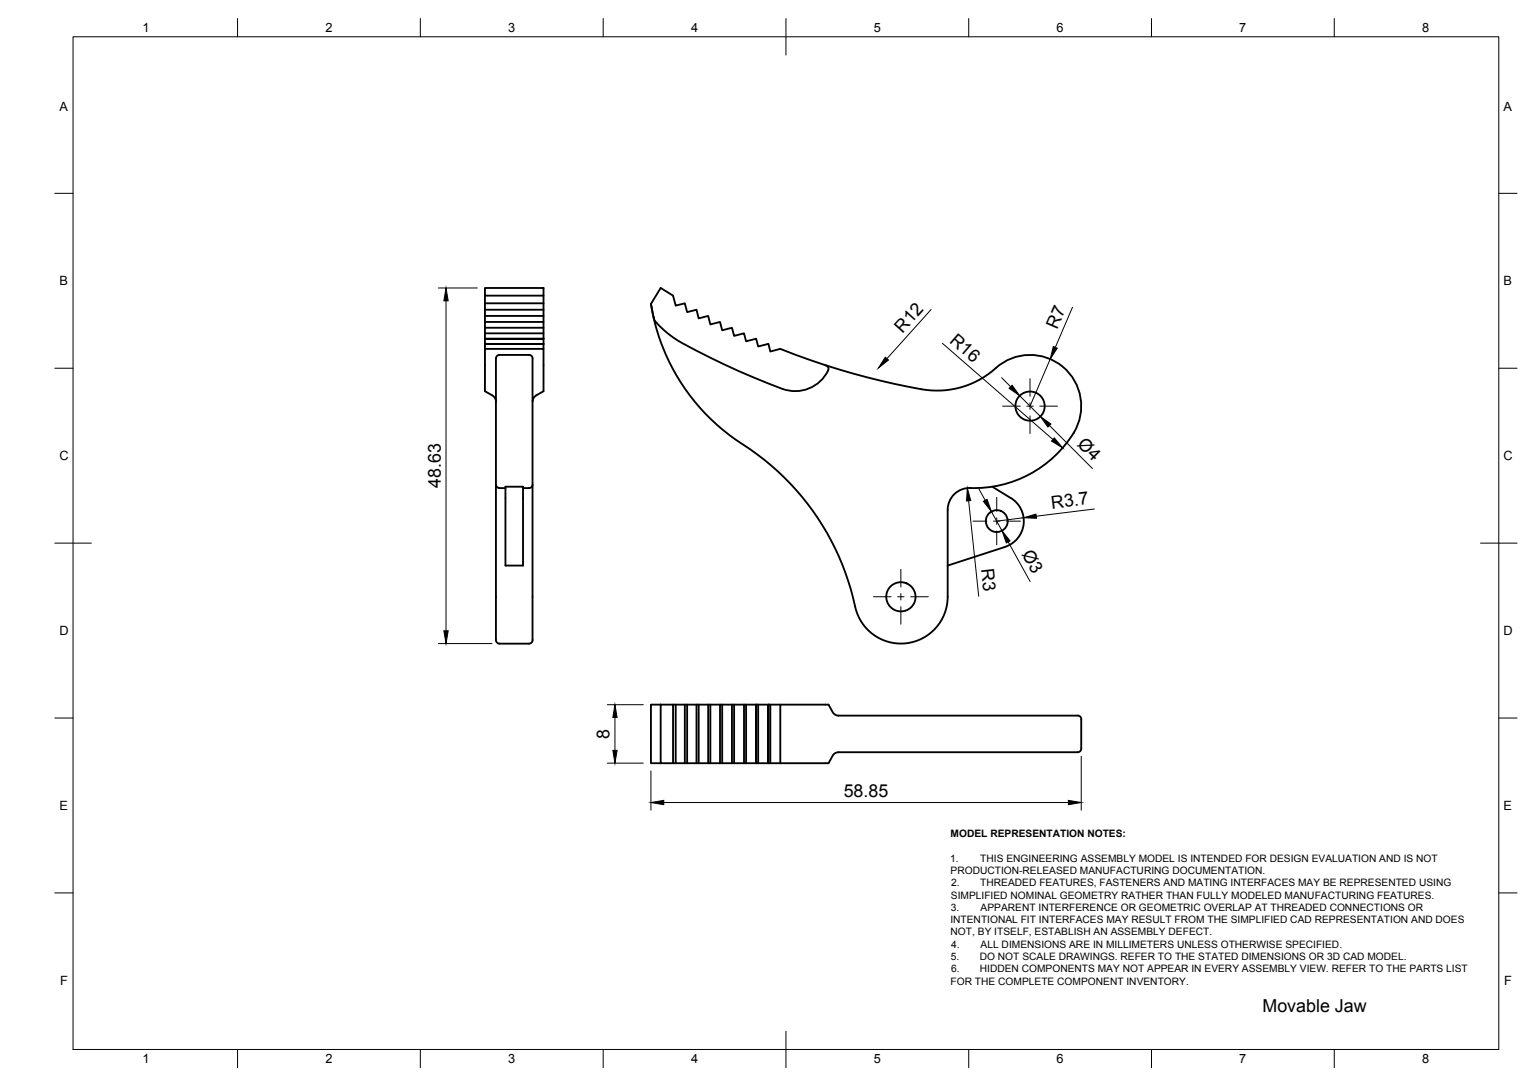
ISO-10303-21;
HEADER;
/* Generated by software containing ST-Developer
 * from STEP Tools, Inc. (www.steptools.com) 
 */

FILE_DESCRIPTION(
/* description */ ('STEP AP214'),
/* implementation_level */ '2;1');

FILE_NAME(
/* name */ 'Movable Jaw.step',
/* time_stamp */ '2026-10-06T11:11:25-07:00',
/* author */ (''),
/* organization */ (''),
/* preprocessor_version */ 'ST-DEVELOPER v20.2',
/* originating_system */ 'Autodesk Translation Framework v15.15.0.0',
/* authorisation */ '');

FILE_SCHEMA (('AUTOMOTIVE_DESIGN { 1 0 10303 214 3 1 1 }'));
ENDSEC;

DATA;
#10=MECHANICAL_DESIGN_GEOMETRIC_PRESENTATION_REPRESENTATION('',(#704),#47717);
#111=ELLIPSE('',#9597,55.9999994580806,27.9999998645779);
#112=ELLIPSE('',#9600,56.0000011433114,28.0000002857322);
#142=CONICAL_SURFACE('',#9608,105.,0.5235987755983);
#143=CONICAL_SURFACE('',#9610,13.5459216391339,0.5235987755983);
#144=CONICAL_SURFACE('',#9612,5.,0.5235987755983);
#145=CONICAL_SURFACE('',#9615,5.,0.5235987755983);
#146=CONICAL_SURFACE('',#9620,13.5459216391339,0.5235987755983);
#147=CONICAL_SURFACE('',#9622,105.,0.5235987755983);
#453=B_SPLINE_CURVE_WITH_KNOTS('',3,(#44399,#44400,#44401,#44402,#44403,
#44404,#44405,#44406,#44407,#44408,#44409,#44410,#44411,#44412,#44413,#44414,
#44415,#44416,#44417,#44418,#44419,#44420,#44421,#44422,#44423,#44424,#44425,
#44426,#44427,#44428,#44429,#44430,#44431,#44432,#44433,#44434,#44435,#44436,
#44437,#44438,#44439,#44440,#44441),.UNSPECIFIED.,.F.,.F.,(4,3,3,3,3,3,
3,3,3,3,3,3,3,3,4),(0.,0.000265218733424361,0.000529943392799562,0.000791311297886273,
0.00104485851075797,0.00120949425781351,0.00140442813951922,0.00159510196316745,
0.00177939478496708,0.00181424138672026,0.00194996928456625,0.00208057934802266,
0.00220782711137267,0.00232952375057779,0.00241898851562701),
 .UNSPECIFIED.);
#454=B_SPLINE_CURVE_WITH_KNOTS('',3,(#44450,#44451,#44452,#44453,#44454,
#44455,#44456,#44457),.UNSPECIFIED.,.F.,.F.,(4,2,2,4),(1.10972417955536E-15,
0.000601563815809569,0.00120312763161803,0.00240625526323496),
 .UNSPECIFIED.);
#455=B_SPLINE_CURVE_WITH_KNOTS('',3,(#44486,#44487,#44488,#44489,#44490,
#44491,#44492,#44493,#44494,#44495,#44496,#44497,#44498,#44499,#44500,#44501,
#44502,#44503,#44504,#44505,#44506,#44507,#44508,#44509,#44510,#44511,#44512,
#44513,#44514,#44515,#44516,#44517,#44518,#44519,#44520,#44521,#44522,#44523,
#44524,#44525),.UNSPECIFIED.,.F.,.F.,(4,3,3,3,3,3,3,3,3,3,3,3,3,4),(0.,
0.000120731756906386,0.000244724286038655,0.000330382072298398,0.00038742395842631,
0.000451543376039767,0.000587355431077626,0.000736422494620045,0.000783140574770168,
0.0007839342580256,0.00111532596981935,0.00117471086215525,0.00117522277660967,
0.00156628114954034),.UNSPECIFIED.);
#456=B_SPLINE_CURVE_WITH_KNOTS('',3,(#44533,#44534,#44535,#44536,#44537,
#44538,#44539,#44540,#44541,#44542,#44543,#44544,#44545,#44546,#44547,#44548,
#44549,#44550,#44551,#44552,#44553,#44554,#44555,#44556,#44557,#44558,#44559,
#44560,#44561,#44562,#44563,#44564,#44565,#44566,#44567,#44568,#44569),
 .UNSPECIFIED.,.F.,.F.,(4,3,3,3,3,3,3,3,3,3,3,3,4),(0.,0.000121030957133445,
0.000244083459183201,0.000368145253824231,0.000391521746120079,0.000542549206905392,
0.000692240215942904,0.000782245350403997,0.000783043492240158,0.0011402076544283,
0.00117391722717013,0.00117456523836024,0.00156608698448032),
 .UNSPECIFIED.);
#457=B_SPLINE_CURVE_WITH_KNOTS('',3,(#44678,#44679,#44680,#44681,#44682,
#44683,#44684),.UNSPECIFIED.,.F.,.F.,(4,3,4),(8.8191888018214E-12,0.00104225234663735,
0.00196541786057149),.UNSPECIFIED.);
#458=B_SPLINE_CURVE_WITH_KNOTS('',3,(#44686,#44687,#44688,#44689,#44690,
#44691,#44692,#44693,#44694,#44695,#44696,#44697,#44698,#44699,#44700,#44701,
#44702,#44703,#44704,#44705,#44706,#44707,#44708,#44709,#44710,#44711,#44712,
#44713,#44714,#44715,#44716),.UNSPECIFIED.,.F.,.F.,(4,3,3,3,3,3,3,3,3,3,
4),(0.,0.000282229008902596,0.000596615472147253,0.000672888082078944,0.000674913983482446,
0.00113908191323505,0.0013477148488729,0.00134982796696489,0.00185411344461373,
0.00236801844152055,0.00269965593392979),.UNSPECIFIED.);
#459=B_SPLINE_CURVE_WITH_KNOTS('',3,(#44724,#44725,#44726,#44727,#44728,
#44729,#44730,#44731,#44732,#44733,#44734,#44735,#44736,#44737,#44738,#44739,
#44740,#44741,#44742,#44743,#44744,#44745,#44746,#44747,#44748,#44749,#44750,
#44751),.UNSPECIFIED.,.F.,.F.,(4,3,3,3,3,3,3,3,3,4),(0.,0.000683898970964164,
0.00134585328061937,0.00134792532155823,0.00179669833308319,0.00201877992092906,
0.0020208379703943,0.00232967550949865,0.00260160458154724,0.00269170656123875),
 .UNSPECIFIED.);
#460=B_SPLINE_CURVE_WITH_KNOTS('',3,(#44753,#44754,#44755,#44756,#44757,
#44758,#44759),.UNSPECIFIED.,.F.,.F.,(4,3,4),(1.55158384577955E-17,0.00104225233782226,
0.0019654178517479),.UNSPECIFIED.);
#461=B_SPLINE_CURVE_WITH_KNOTS('',3,(#44766,#44767,#44768,#44769,#44770,
#44771,#44772,#44773,#44774,#44775,#44776,#44777),.UNSPECIFIED.,.F.,.F.,
(4,2,2,2,2,4),(0.,0.023927482322817,0.0451601219442732,0.0651153892897719,
0.0785588651844482,0.0909362631271192),.UNSPECIFIED.);
#462=B_SPLINE_CURVE_WITH_KNOTS('',3,(#44785,#44786,#44787,#44788,#44789,
#44790),.UNSPECIFIED.,.F.,.F.,(4,2,4),(1.03628274237769E-6,0.0204474690808872,
0.0408541618075523),.UNSPECIFIED.);
#463=B_SPLINE_CURVE_WITH_KNOTS('',3,(#44831,#44832,#44833,#44834),
 .UNSPECIFIED.,.F.,.F.,(4,4),(0.,0.00159208620889079),.UNSPECIFIED.);
#464=B_SPLINE_CURVE_WITH_KNOTS('',3,(#44836,#44837,#44838,#44839,#44840,
#44841),.UNSPECIFIED.,.F.,.F.,(4,2,4),(-0.0108288738373355,-0.00541184520716738,
0.),.UNSPECIFIED.);
#465=B_SPLINE_CURVE_WITH_KNOTS('',3,(#44857,#44858,#44859,#44860,#44861,
#44862),.UNSPECIFIED.,.F.,.F.,(4,2,4),(-0.0108279843969241,-0.00541695432919009,
-7.41619925991033E-7),.UNSPECIFIED.);
#466=B_SPLINE_CURVE_WITH_KNOTS('',3,(#44868,#44869,#44870,#44871),
 .UNSPECIFIED.,.F.,.F.,(4,4),(1.72172026516128E-9,0.00159208793060872),
 .UNSPECIFIED.);
#467=B_SPLINE_CURVE_WITH_KNOTS('',3,(#44877,#44878,#44879,#44880,#44881,
#44882,#44883,#44884,#44885,#44886,#44887,#44888),.UNSPECIFIED.,.F.,.F.,
(4,2,2,2,2,4),(-0.0909372297788789,-0.0786310994776589,-0.0652694224322856,
-0.0453380124663928,-0.0241275039307517,0.),.UNSPECIFIED.);
#468=B_SPLINE_CURVE_WITH_KNOTS('',3,(#44922,#44923,#44924,#44925,#44926,
#44927),.UNSPECIFIED.,.F.,.F.,(4,2,4),(-0.0408541865438099,-0.0204437555046671,
-1.03628388816493E-6),.UNSPECIFIED.);
#469=B_SPLINE_CURVE_WITH_KNOTS('',3,(#44929,#44930,#44931,#44932,#44933,
#44934,#44935,#44936,#44937,#44938,#44939,#44940,#44941,#44942,#44943,#44944,
#44945,#44946,#44947,#44948,#44949,#44950,#44951,#44952,#44953,#44954,#44955,
#44956,#44957,#44958,#44959,#44960,#44961,#44962),.UNSPECIFIED.,.F.,.F.,
(4,3,3,3,3,3,3,3,3,3,3,4),(0.,0.000262944884148408,0.000263234297577755,
0.000494857606554129,0.000525889768296816,0.000526476175615979,0.00064121097647369,
0.000757086494550119,0.000788834652445224,0.000880494124966269,0.000970158609493951,
0.00105177953659363),.UNSPECIFIED.);
#470=B_SPLINE_CURVE_WITH_KNOTS('',3,(#44966,#44967,#44968,#44969,#44970,
#44971,#44972,#44973,#44974,#44975,#44976,#44977,#44978,#44979,#44980,#44981,
#44982,#44983,#44984,#44985,#44986,#44987,#44988,#44989,#44990,#44991,#44992,
#44993,#44994,#44995,#44996,#44997,#44998,#44999,#45000,#45001,#45002),
 .UNSPECIFIED.,.F.,.F.,(4,3,3,3,3,3,3,3,3,3,3,3,4),(0.,0.000244362774360397,
0.000262384380603159,0.000262964527186242,0.000497872683618592,0.0005253349756591,
0.000525929054372485,0.000639225228153213,0.000753740945662581,0.000788893581558727,
0.000881307299681151,0.000971994008335542,0.00105185810874497),
 .UNSPECIFIED.);
#590=(
BOUNDED_SURFACE()
B_SPLINE_SURFACE(3,2,((#45068,#45069,#45070),(#45071,#45072,#45073),(#45074,
#45075,#45076),(#45077,#45078,#45079),(#45080,#45081,#45082),(#45083,#45084,
#45085),(#45086,#45087,#45088),(#45089,#45090,#45091)),.UNSPECIFIED.,.F.,
 .F.,.F.)
B_SPLINE_SURFACE_WITH_KNOTS((4,2,2,4),(3,3),(-0.000265671039808014,0.000664177599544138,
0.00132835519908425,0.00292238143798051),(-0.000697566251991853,1.),
 .UNSPECIFIED.)
GEOMETRIC_REPRESENTATION_ITEM()
RATIONAL_B_SPLINE_SURFACE(((1.00006735358899,0.951722442998278,1.),(1.00009085795633,
0.934875034398606,1.),(1.00011995255585,0.914020671505109,1.),(1.00017679132716,
0.873279902332299,1.),(1.000202236158,0.855041612592702,1.),(1.00029314270923,
0.789881815244371,1.),(1.00036608854593,0.737595859260726,1.),(1.00044993425484,
0.677497116903894,1.)))
REPRESENTATION_ITEM('')
SURFACE()
);
#591=(
BOUNDED_SURFACE()
B_SPLINE_SURFACE(3,2,((#45093,#45094,#45095),(#45096,#45097,#45098),(#45099,
#45100,#45101),(#45102,#45103,#45104)),.UNSPECIFIED.,.F.,.F.,.F.)
B_SPLINE_SURFACE_WITH_KNOTS((4,4),(3,3),(1.73472347597681E-18,0.00194751686681009),
(0.,1.),.UNSPECIFIED.)
GEOMETRIC_REPRESENTATION_ITEM()
RATIONAL_B_SPLINE_SURFACE(((1.,0.9363704575632,1.),(1.,0.937911573932337,
1.),(1.,0.939551224752395,1.),(1.,0.941276432107511,1.)))
REPRESENTATION_ITEM('')
SURFACE()
);
#592=(
BOUNDED_SURFACE()
B_SPLINE_SURFACE(3,2,((#45115,#45116,#45117),(#45118,#45119,#45120),(#45121,
#45122,#45123),(#45124,#45125,#45126),(#45127,#45128,#45129),(#45130,#45131,
#45132),(#45133,#45134,#45135),(#45136,#45137,#45138)),.UNSPECIFIED.,.F.,
 .F.,.F.)
B_SPLINE_SURFACE_WITH_KNOTS((4,2,2,4),(3,3),(-0.000264848297699882,0.00132424148849942,
0.00198636223274913,0.00291333127469873),(-0.000376747913465724,1.),
 .UNSPECIFIED.)
GEOMETRIC_REPRESENTATION_ITEM()
RATIONAL_B_SPLINE_SURFACE(((1.00024295987203,0.677556446441725,1.),(1.00019753111789,
0.73784709770907,1.),(1.00015862247899,0.789484595236775,1.),(1.00010910533939,
0.855201136507422,1.),(1.00009527454653,0.873556636784662,1.),(1.00006486797912,
0.91391063254542,1.),(1.00004913297578,0.934793300746539,1.),(1.0000362266027,
0.951921959744005,1.)))
REPRESENTATION_ITEM('')
SURFACE()
);
#593=(
BOUNDED_SURFACE()
B_SPLINE_SURFACE(3,2,((#45140,#45141,#45142),(#45143,#45144,#45145),(#45146,
#45147,#45148),(#45149,#45150,#45151)),.UNSPECIFIED.,.F.,.F.,.F.)
B_SPLINE_SURFACE_WITH_KNOTS((4,4),(3,3),(-3.46944695195361E-18,0.00194751686680595),
(0.,1.),.UNSPECIFIED.)
GEOMETRIC_REPRESENTATION_ITEM()
RATIONAL_B_SPLINE_SURFACE(((1.,0.936370457563209,1.),(1.,0.937911573932344,
1.),(1.,0.939551224752402,1.),(1.,0.941276432107508,1.)))
REPRESENTATION_ITEM('')
SURFACE()
);
#594=(
BOUNDED_SURFACE()
B_SPLINE_SURFACE(3,2,((#45152,#45153,#45154),(#45155,#45156,#45157),(#45158,
#45159,#45160),(#45161,#45162,#45163)),.UNSPECIFIED.,.F.,.F.,.F.)
B_SPLINE_SURFACE_WITH_KNOTS((4,4),(3,3),(-8.67361737988404E-19,0.00145502531726256),
(0.,1.),.UNSPECIFIED.)
GEOMETRIC_REPRESENTATION_ITEM()
RATIONAL_B_SPLINE_SURFACE(((1.,0.668532680377463,1.),(1.,0.667444009600454,
1.),(1.,0.666151431295988,1.),(1.,0.66453110293118,1.)))
REPRESENTATION_ITEM('')
SURFACE()
);
#595=(
BOUNDED_SURFACE()
B_SPLINE_SURFACE(3,2,((#45165,#45166,#45167),(#45168,#45169,#45170),(#45171,
#45172,#45173),(#45174,#45175,#45176),(#45177,#45178,#45179),(#45180,#45181,
#45182),(#45183,#45184,#45185),(#45186,#45187,#45188)),.UNSPECIFIED.,.F.,
 .F.,.F.)
B_SPLINE_SURFACE_WITH_KNOTS((4,2,2,4),(3,3),(-8.23993651088983E-18,0.000785858548320119,
0.00117878782248018,0.00157171709664025),(0.,1.),.UNSPECIFIED.)
GEOMETRIC_REPRESENTATION_ITEM()
RATIONAL_B_SPLINE_SURFACE(((1.,0.707106781186552,1.),(1.,0.700392709855563,
1.),(1.,0.693103478140052,1.),(1.,0.68292873029758,1.),(1.,0.679593975234355,
1.),(1.,0.673572573507934,1.),(1.,0.670859596930162,1.),(1.,0.668532680377463,
1.)))
REPRESENTATION_ITEM('')
SURFACE()
);
#596=(
BOUNDED_SURFACE()
B_SPLINE_SURFACE(3,2,((#45208,#45209,#45210),(#45211,#45212,#45213),(#45214,
#45215,#45216),(#45217,#45218,#45219),(#45220,#45221,#45222),(#45223,#45224,
#45225),(#45226,#45227,#45228),(#45229,#45230,#45231)),.UNSPECIFIED.,.F.,
 .F.,.F.)
B_SPLINE_SURFACE_WITH_KNOTS((4,2,2,4),(3,3),(-1.25767452008319E-17,0.000785889192074472,
0.00117883378811171,0.00157177838414896),(0.,1.),.UNSPECIFIED.)
GEOMETRIC_REPRESENTATION_ITEM()
RATIONAL_B_SPLINE_SURFACE(((1.,0.668532680377451,1.),(1.,0.673123216892149,
1.),(1.,0.679555858731309,1.),(1.,0.68973495589728,1.),(1.,0.693295125056467,
1.),(1.,0.700263684314459,1.),(1.,0.703699964289598,1.),(1.,0.707106781186548,
1.)))
REPRESENTATION_ITEM('')
SURFACE()
);
#597=(
BOUNDED_SURFACE()
B_SPLINE_SURFACE(3,2,((#45233,#45234,#45235),(#45236,#45237,#45238),(#45239,
#45240,#45241),(#45242,#45243,#45244)),.UNSPECIFIED.,.F.,.F.,.F.)
B_SPLINE_SURFACE_WITH_KNOTS((4,4),(3,3),(-8.67361737988404E-19,0.00145502531726205),
(0.,1.),.UNSPECIFIED.)
GEOMETRIC_REPRESENTATION_ITEM()
RATIONAL_B_SPLINE_SURFACE(((1.,0.668532680377451,1.),(1.,0.667444009600447,
1.),(1.,0.666151431295967,1.),(1.,0.664531102931197,1.)))
REPRESENTATION_ITEM('')
SURFACE()
);
#630=TOROIDAL_SURFACE('',#9516,5.9,0.5);
#631=TOROIDAL_SURFACE('',#9521,5.9,0.5);
#632=TOROIDAL_SURFACE('',#9535,14.989297312108,1.);
#633=TOROIDAL_SURFACE('',#9539,14.989297312108,1.);
#634=TOROIDAL_SURFACE('',#9626,6.44337567297407,1.);
#635=TOROIDAL_SURFACE('',#9628,106.443375672974,1.);
#636=TOROIDAL_SURFACE('',#9629,6.44337567297407,1.);
#637=TOROIDAL_SURFACE('',#9631,106.443375672974,1.);
#638=TOROIDAL_SURFACE('',#9660,15.5,0.5);
#639=TOROIDAL_SURFACE('',#9663,3.5,0.5);
#640=TOROIDAL_SURFACE('',#9666,35.5,0.5);
#641=TOROIDAL_SURFACE('',#9668,27.5,0.5);
#642=TOROIDAL_SURFACE('',#9671,15.5,0.5);
#643=TOROIDAL_SURFACE('',#9674,3.5,0.5);
#644=TOROIDAL_SURFACE('',#9677,35.5,0.5);
#645=TOROIDAL_SURFACE('',#9679,27.5,0.5);
#646=TOROIDAL_SURFACE('',#9684,100.5,0.5);
#647=TOROIDAL_SURFACE('',#9686,12.5,0.5);
#648=TOROIDAL_SURFACE('',#9688,6.5,0.5);
#649=TOROIDAL_SURFACE('',#9696,6.5,0.5);
#650=TOROIDAL_SURFACE('',#9698,12.5,0.5);
#651=TOROIDAL_SURFACE('',#9700,100.5,0.5);
#680=SHAPE_REPRESENTATION_RELATIONSHIP('SRR','None',#47767,#692);
#692=ADVANCED_BREP_SHAPE_REPRESENTATION('',(#716),#47711);
#704=STYLED_ITEM('',(#47830),#716);
#716=MANIFOLD_SOLID_BREP('Body1',#8931);
#731=FACE_BOUND('',#2898,.T.);
#732=FACE_BOUND('',#2899,.T.);
#733=FACE_BOUND('',#2901,.T.);
#734=FACE_BOUND('',#2902,.T.);
#735=FACE_BOUND('',#2927,.T.);
#736=FACE_BOUND('',#2929,.T.);
#812=PLANE('',#9563);
#813=PLANE('',#9573);
#814=PLANE('',#9583);
#815=PLANE('',#9595);
#816=PLANE('',#9604);
#817=PLANE('',#9611);
#818=PLANE('',#9619);
#819=PLANE('',#9625);
#820=PLANE('',#9635);
#821=PLANE('',#9636);
#822=PLANE('',#9638);
#823=PLANE('',#9641);
#824=PLANE('',#9642);
#825=PLANE('',#9643);
#826=PLANE('',#9644);
#827=PLANE('',#9645);
#828=PLANE('',#9646);
#829=PLANE('',#9647);
#830=PLANE('',#9648);
#831=PLANE('',#9649);
#832=PLANE('',#9650);
#833=PLANE('',#9651);
#834=PLANE('',#9652);
#835=PLANE('',#9653);
#836=PLANE('',#9654);
#837=PLANE('',#9655);
#838=PLANE('',#9656);
#839=PLANE('',#9657);
#840=PLANE('',#9658);
#841=PLANE('',#9659);
#1146=LINE('',#44377,#1633);
#1147=LINE('',#44383,#1634);
#1148=LINE('',#44389,#1635);
#1149=LINE('',#44463,#1636);
#1150=LINE('',#44466,#1637);
#1151=LINE('',#44468,#1638);
#1152=LINE('',#44469,#1639);
#1153=LINE('',#44475,#1640);
#1154=LINE('',#44478,#1641);
#1155=LINE('',#44529,#1642);
#1156=LINE('',#44574,#1643);
#1157=LINE('',#44580,#1644);
#1158=LINE('',#44583,#1645);
#1159=LINE('',#44587,#1646);
#1160=LINE('',#44591,#1647);
#1161=LINE('',#44606,#1648);
#1162=LINE('',#44622,#1649);
#1163=LINE('',#44632,#1650);
#1164=LINE('',#44634,#1651);
#1165=LINE('',#44636,#1652);
#1166=LINE('',#44638,#1653);
#1167=LINE('',#44640,#1654);
#1168=LINE('',#44641,#1655);
#1169=LINE('',#44646,#1656);
#1170=LINE('',#44650,#1657);
#1171=LINE('',#44654,#1658);
#1172=LINE('',#44659,#1659);
#1173=LINE('',#44663,#1660);
#1174=LINE('',#44670,#1661);
#1175=LINE('',#44672,#1662);
#1176=LINE('',#44673,#1663);
#1177=LINE('',#44720,#1664);
#1178=LINE('',#44791,#1665);
#1179=LINE('',#44793,#1666);
#1180=LINE('',#44795,#1667);
#1181=LINE('',#44797,#1668);
#1182=LINE('',#44799,#1669);
#1183=LINE('',#44801,#1670);
#1184=LINE('',#44803,#1671);
#1185=LINE('',#44805,#1672);
#1186=LINE('',#44807,#1673);
#1187=LINE('',#44809,#1674);
#1188=LINE('',#44811,#1675);
#1189=LINE('',#44813,#1676);
#1190=LINE('',#44815,#1677);
#1191=LINE('',#44817,#1678);
#1192=LINE('',#44818,#1679);
#1193=LINE('',#44820,#1680);
#1194=LINE('',#44821,#1681);
#1195=LINE('',#44823,#1682);
#1196=LINE('',#44824,#1683);
#1197=LINE('',#44827,#1684);
#1198=LINE('',#44829,#1685);
#1199=LINE('',#44854,#1686);
#1200=LINE('',#44863,#1687);
#1201=LINE('',#44872,#1688);
#1202=LINE('',#44890,#1689);
#1203=LINE('',#44891,#1690);
#1204=LINE('',#44893,#1691);
#1205=LINE('',#44894,#1692);
#1206=LINE('',#44896,#1693);
#1207=LINE('',#44898,#1694);
#1208=LINE('',#44900,#1695);
#1209=LINE('',#44902,#1696);
#1210=LINE('',#44904,#1697);
#1211=LINE('',#44906,#1698);
#1212=LINE('',#44908,#1699);
#1213=LINE('',#44910,#1700);
#1214=LINE('',#44912,#1701);
#1215=LINE('',#44914,#1702);
#1216=LINE('',#44916,#1703);
#1217=LINE('',#44918,#1704);
#1218=LINE('',#44920,#1705);
#1219=LINE('',#44921,#1706);
#1220=LINE('',#45010,#1707);
#1221=LINE('',#45012,#1708);
#1222=LINE('',#45013,#1709);
#1223=LINE('',#45016,#1710);
#1224=LINE('',#45021,#1711);
#1225=LINE('',#45023,#1712);
#1226=LINE('',#45026,#1713);
#1227=LINE('',#45027,#1714);
#1228=LINE('',#45030,#1715);
#1229=LINE('',#45032,#1716);
#1230=LINE('',#45033,#1717);
#1231=LINE('',#45035,#1718);
#1232=LINE('',#45036,#1719);
#1233=LINE('',#45038,#1720);
#1234=LINE('',#45039,#1721);
#1235=LINE('',#45041,#1722);
#1236=LINE('',#45042,#1723);
#1237=LINE('',#45044,#1724);
#1238=LINE('',#45045,#1725);
#1239=LINE('',#45053,#1726);
#1240=LINE('',#45056,#1727);
#1633=VECTOR('',#11135,1.5);
#1634=VECTOR('',#11142,2.00000000000001);
#1635=VECTOR('',#11149,2.);
#1636=VECTOR('',#11172,1000.);
#1637=VECTOR('',#11175,1000.);
#1638=VECTOR('',#11178,1000.);
#1639=VECTOR('',#11179,1000.);
#1640=VECTOR('',#11184,1000.);
#1641=VECTOR('',#11187,1000.);
#1642=VECTOR('',#11196,1000.);
#1643=VECTOR('',#11203,1000.);
#1644=VECTOR('',#11208,1000.);
#1645=VECTOR('',#11211,1000.);
#1646=VECTOR('',#11214,1000.);
#1647=VECTOR('',#11217,1000.);
#1648=VECTOR('',#11234,1000.);
#1649=VECTOR('',#11251,1000.);
#1650=VECTOR('',#11264,1000.);
#1651=VECTOR('',#11265,1000.);
#1652=VECTOR('',#11266,1000.);
#1653=VECTOR('',#11267,1000.);
#1654=VECTOR('',#11268,1000.);
#1655=VECTOR('',#11269,1000.);
#1656=VECTOR('',#11274,1000.);
#1657=VECTOR('',#11277,1000.);
#1658=VECTOR('',#11280,1000.);
#1659=VECTOR('',#11285,1000.);
#1660=VECTOR('',#11288,1000.);
#1661=VECTOR('',#11299,1000.);
#1662=VECTOR('',#11300,1000.);
#1663=VECTOR('',#11301,1000.);
#1664=VECTOR('',#11308,1000.);
#1665=VECTOR('',#11327,1000.);
#1666=VECTOR('',#11328,1000.);
#1667=VECTOR('',#11329,1000.);
#1668=VECTOR('',#11330,1000.);
#1669=VECTOR('',#11331,1000.);
#1670=VECTOR('',#11332,1000.);
#1671=VECTOR('',#11333,1000.);
#1672=VECTOR('',#11334,1000.);
#1673=VECTOR('',#11335,1000.);
#1674=VECTOR('',#11336,1000.);
#1675=VECTOR('',#11337,1000.);
#1676=VECTOR('',#11338,1000.);
#1677=VECTOR('',#11339,1000.);
#1678=VECTOR('',#11340,1000.);
#1679=VECTOR('',#11341,1000.);
#1680=VECTOR('',#11342,1000.);
#1681=VECTOR('',#11343,1000.);
#1682=VECTOR('',#11344,1000.);
#1683=VECTOR('',#11345,1000.);
#1684=VECTOR('',#11348,1000.);
#1685=VECTOR('',#11351,1000.);
#1686=VECTOR('',#11370,1000.);
#1687=VECTOR('',#11373,1000.);
#1688=VECTOR('',#11378,1000.);
#1689=VECTOR('',#11387,1000.);
#1690=VECTOR('',#11388,1000.);
#1691=VECTOR('',#11389,1000.);
#1692=VECTOR('',#11390,1000.);
#1693=VECTOR('',#11391,1000.);
#1694=VECTOR('',#11392,1000.);
#1695=VECTOR('',#11393,1000.);
#1696=VECTOR('',#11394,1000.);
#1697=VECTOR('',#11395,1000.);
#1698=VECTOR('',#11396,1000.);
#1699=VECTOR('',#11397,1000.);
#1700=VECTOR('',#11398,1000.);
#1701=VECTOR('',#11399,1000.);
#1702=VECTOR('',#11400,1000.);
#1703=VECTOR('',#11401,1000.);
#1704=VECTOR('',#11402,1000.);
#1705=VECTOR('',#11403,1000.);
#1706=VECTOR('',#11404,1000.);
#1707=VECTOR('',#11425,1000.);
#1708=VECTOR('',#11426,1000.);
#1709=VECTOR('',#11427,1000.);
#1710=VECTOR('',#11430,1000.);
#1711=VECTOR('',#11437,1000.);
#1712=VECTOR('',#11440,1000.);
#1713=VECTOR('',#11445,1000.);
#1714=VECTOR('',#11446,1000.);
#1715=VECTOR('',#11451,1000.);
#1716=VECTOR('',#11454,1000.);
#1717=VECTOR('',#11455,1000.);
#1718=VECTOR('',#11458,1000.);
#1719=VECTOR('',#11459,1000.);
#1720=VECTOR('',#11462,1000.);
#1721=VECTOR('',#11463,1000.);
#1722=VECTOR('',#11466,1000.);
#1723=VECTOR('',#11467,1000.);
#1724=VECTOR('',#11470,1000.);
#1725=VECTOR('',#11471,1000.);
#1726=VECTOR('',#11486,1000.);
#1727=VECTOR('',#11491,1000.);
#1998=CYLINDRICAL_SURFACE('',#9526,1.5);
#1999=CYLINDRICAL_SURFACE('',#9529,2.00000000000001);
#2000=CYLINDRICAL_SURFACE('',#9532,2.);
#2001=CYLINDRICAL_SURFACE('',#9543,100.);
#2002=CYLINDRICAL_SURFACE('',#9546,6.4);
#2003=CYLINDRICAL_SURFACE('',#9547,100.);
#2004=CYLINDRICAL_SURFACE('',#9550,100.);
#2005=CYLINDRICAL_SURFACE('',#9557,100.);
#2006=CYLINDRICAL_SURFACE('',#9560,3.);
#2007=CYLINDRICAL_SURFACE('',#9584,16.);
#2008=CYLINDRICAL_SURFACE('',#9589,7.);
#2009=CYLINDRICAL_SURFACE('',#9592,12.);
#2010=CYLINDRICAL_SURFACE('',#9596,28.);
#2011=CYLINDRICAL_SURFACE('',#9601,35.);
#2012=CYLINDRICAL_SURFACE('',#9632,3.);
#2013=CYLINDRICAL_SURFACE('',#9640,3.7);
#2014=CYLINDRICAL_SURFACE('',#9665,0.500000000000001);
#2015=CYLINDRICAL_SURFACE('',#9676,0.500000000000001);
#2016=CYLINDRICAL_SURFACE('',#9692,0.499999999999999);
#2363=FACE_OUTER_BOUND('',#2884,.T.);
#2364=FACE_OUTER_BOUND('',#2885,.T.);
#2365=FACE_OUTER_BOUND('',#2886,.T.);
#2366=FACE_OUTER_BOUND('',#2887,.T.);
#2367=FACE_OUTER_BOUND('',#2888,.T.);
#2368=FACE_OUTER_BOUND('',#2889,.T.);
#2369=FACE_OUTER_BOUND('',#2890,.T.);
#2370=FACE_OUTER_BOUND('',#2891,.T.);
#2371=FACE_OUTER_BOUND('',#2892,.T.);
#2372=FACE_OUTER_BOUND('',#2893,.T.);
#2373=FACE_OUTER_BOUND('',#2894,.T.);
#2374=FACE_OUTER_BOUND('',#2895,.T.);
#2375=FACE_OUTER_BOUND('',#2896,.T.);
#2376=FACE_OUTER_BOUND('',#2897,.T.);
#2377=FACE_OUTER_BOUND('',#2900,.T.);
#2378=FACE_OUTER_BOUND('',#2903,.T.);
#2379=FACE_OUTER_BOUND('',#2904,.T.);
#2380=FACE_OUTER_BOUND('',#2905,.T.);
#2381=FACE_OUTER_BOUND('',#2906,.T.);
#2382=FACE_OUTER_BOUND('',#2907,.T.);
#2383=FACE_OUTER_BOUND('',#2908,.T.);
#2384=FACE_OUTER_BOUND('',#2909,.T.);
#2385=FACE_OUTER_BOUND('',#2910,.T.);
#2386=FACE_OUTER_BOUND('',#2911,.T.);
#2387=FACE_OUTER_BOUND('',#2912,.T.);
#2388=FACE_OUTER_BOUND('',#2913,.T.);
#2389=FACE_OUTER_BOUND('',#2914,.T.);
#2390=FACE_OUTER_BOUND('',#2915,.T.);
#2391=FACE_OUTER_BOUND('',#2916,.T.);
#2392=FACE_OUTER_BOUND('',#2917,.T.);
#2393=FACE_OUTER_BOUND('',#2918,.T.);
#2394=FACE_OUTER_BOUND('',#2919,.T.);
#2395=FACE_OUTER_BOUND('',#2920,.T.);
#2396=FACE_OUTER_BOUND('',#2921,.T.);
#2397=FACE_OUTER_BOUND('',#2922,.T.);
#2398=FACE_OUTER_BOUND('',#2923,.T.);
#2399=FACE_OUTER_BOUND('',#2924,.T.);
#2400=FACE_OUTER_BOUND('',#2925,.T.);
#2401=FACE_OUTER_BOUND('',#2926,.T.);
#2402=FACE_OUTER_BOUND('',#2928,.T.);
#2403=FACE_OUTER_BOUND('',#2930,.T.);
#2404=FACE_OUTER_BOUND('',#2931,.T.);
#2405=FACE_OUTER_BOUND('',#2932,.T.);
#2406=FACE_OUTER_BOUND('',#2933,.T.);
#2407=FACE_OUTER_BOUND('',#2934,.T.);
#2408=FACE_OUTER_BOUND('',#2935,.T.);
#2409=FACE_OUTER_BOUND('',#2936,.T.);
#2410=FACE_OUTER_BOUND('',#2937,.T.);
#2411=FACE_OUTER_BOUND('',#2938,.T.);
#2412=FACE_OUTER_BOUND('',#2939,.T.);
#2413=FACE_OUTER_BOUND('',#2940,.T.);
#2414=FACE_OUTER_BOUND('',#2941,.T.);
#2415=FACE_OUTER_BOUND('',#2942,.T.);
#2416=FACE_OUTER_BOUND('',#2943,.T.);
#2417=FACE_OUTER_BOUND('',#2944,.T.);
#2418=FACE_OUTER_BOUND('',#2945,.T.);
#2419=FACE_OUTER_BOUND('',#2946,.T.);
#2420=FACE_OUTER_BOUND('',#2947,.T.);
#2421=FACE_OUTER_BOUND('',#2948,.T.);
#2422=FACE_OUTER_BOUND('',#2949,.T.);
#2423=FACE_OUTER_BOUND('',#2950,.T.);
#2424=FACE_OUTER_BOUND('',#2951,.T.);
#2425=FACE_OUTER_BOUND('',#2952,.T.);
#2426=FACE_OUTER_BOUND('',#2953,.T.);
#2427=FACE_OUTER_BOUND('',#2954,.T.);
#2428=FACE_OUTER_BOUND('',#2955,.T.);
#2429=FACE_OUTER_BOUND('',#2956,.T.);
#2430=FACE_OUTER_BOUND('',#2957,.T.);
#2431=FACE_OUTER_BOUND('',#2958,.T.);
#2432=FACE_OUTER_BOUND('',#2959,.T.);
#2433=FACE_OUTER_BOUND('',#2960,.T.);
#2434=FACE_OUTER_BOUND('',#2961,.T.);
#2435=FACE_OUTER_BOUND('',#2962,.T.);
#2436=FACE_OUTER_BOUND('',#2963,.T.);
#2437=FACE_OUTER_BOUND('',#2964,.T.);
#2438=FACE_OUTER_BOUND('',#2965,.T.);
#2439=FACE_OUTER_BOUND('',#2966,.T.);
#2440=FACE_OUTER_BOUND('',#2967,.T.);
#2441=FACE_OUTER_BOUND('',#2968,.T.);
#2442=FACE_OUTER_BOUND('',#2969,.T.);
#2443=FACE_OUTER_BOUND('',#2970,.T.);
#2444=FACE_OUTER_BOUND('',#2971,.T.);
#2445=FACE_OUTER_BOUND('',#2972,.T.);
#2446=FACE_OUTER_BOUND('',#2973,.T.);
#2447=FACE_OUTER_BOUND('',#2974,.T.);
#2448=FACE_OUTER_BOUND('',#2975,.T.);
#2449=FACE_OUTER_BOUND('',#2976,.T.);
#2884=EDGE_LOOP('',(#7347,#7348,#7349,#7350));
#2885=EDGE_LOOP('',(#7351,#7352,#7353,#7354));
#2886=EDGE_LOOP('',(#7355,#7356,#7357,#7358));
#2887=EDGE_LOOP('',(#7359,#7360,#7361,#7362));
#2888=EDGE_LOOP('',(#7363,#7364,#7365,#7366));
#2889=EDGE_LOOP('',(#7367,#7368,#7369,#7370));
#2890=EDGE_LOOP('',(#7371,#7372,#7373,#7374));
#2891=EDGE_LOOP('',(#7375,#7376,#7377,#7378));
#2892=EDGE_LOOP('',(#7379,#7380,#7381,#7382));
#2893=EDGE_LOOP('',(#7383,#7384,#7385,#7386));
#2894=EDGE_LOOP('',(#7387,#7388,#7389,#7390,#7391,#7392,#7393,#7394,#7395,
#7396));
#2895=EDGE_LOOP('',(#7397,#7398,#7399,#7400));
#2896=EDGE_LOOP('',(#7401,#7402,#7403,#7404));
#2897=EDGE_LOOP('',(#7405,#7406,#7407,#7408,#7409,#7410,#7411,#7412,#7413,
#7414,#7415,#7416));
#2898=EDGE_LOOP('',(#7417));
#2899=EDGE_LOOP('',(#7418));
#2900=EDGE_LOOP('',(#7419,#7420,#7421,#7422,#7423,#7424,#7425,#7426,#7427,
#7428,#7429,#7430));
#2901=EDGE_LOOP('',(#7431));
#2902=EDGE_LOOP('',(#7432));
#2903=EDGE_LOOP('',(#7433,#7434,#7435,#7436,#7437,#7438,#7439,#7440));
#2904=EDGE_LOOP('',(#7441,#7442,#7443,#7444,#7445,#7446,#7447,#7448));
#2905=EDGE_LOOP('',(#7449,#7450,#7451,#7452));
#2906=EDGE_LOOP('',(#7453,#7454,#7455,#7456));
#2907=EDGE_LOOP('',(#7457,#7458,#7459,#7460));
#2908=EDGE_LOOP('',(#7461,#7462,#7463,#7464,#7465,#7466,#7467,#7468,#7469,
#7470));
#2909=EDGE_LOOP('',(#7471,#7472,#7473,#7474));
#2910=EDGE_LOOP('',(#7475,#7476,#7477,#7478,#7479,#7480,#7481,#7482,#7483,
#7484,#7485,#7486,#7487,#7488,#7489,#7490,#7491,#7492,#7493,#7494,#7495,
#7496,#7497,#7498,#7499,#7500,#7501,#7502,#7503));
#2911=EDGE_LOOP('',(#7504,#7505,#7506,#7507));
#2912=EDGE_LOOP('',(#7508,#7509,#7510,#7511));
#2913=EDGE_LOOP('',(#7512,#7513,#7514));
#2914=EDGE_LOOP('',(#7515,#7516,#7517,#7518));
#2915=EDGE_LOOP('',(#7519,#7520,#7521,#7522));
#2916=EDGE_LOOP('',(#7523,#7524,#7525));
#2917=EDGE_LOOP('',(#7526,#7527,#7528,#7529));
#2918=EDGE_LOOP('',(#7530,#7531,#7532,#7533));
#2919=EDGE_LOOP('',(#7534,#7535,#7536,#7537,#7538,#7539,#7540,#7541,#7542,
#7543,#7544,#7545,#7546,#7547,#7548,#7549,#7550,#7551,#7552,#7553,#7554,
#7555,#7556,#7557,#7558,#7559,#7560,#7561,#7562));
#2920=EDGE_LOOP('',(#7563,#7564,#7565,#7566));
#2921=EDGE_LOOP('',(#7567,#7568,#7569,#7570));
#2922=EDGE_LOOP('',(#7571,#7572,#7573,#7574));
#2923=EDGE_LOOP('',(#7575,#7576,#7577,#7578));
#2924=EDGE_LOOP('',(#7579,#7580,#7581,#7582));
#2925=EDGE_LOOP('',(#7583,#7584,#7585,#7586));
#2926=EDGE_LOOP('',(#7587,#7588,#7589,#7590,#7591,#7592));
#2927=EDGE_LOOP('',(#7593));
#2928=EDGE_LOOP('',(#7594,#7595,#7596,#7597,#7598,#7599));
#2929=EDGE_LOOP('',(#7600));
#2930=EDGE_LOOP('',(#7601,#7602,#7603,#7604));
#2931=EDGE_LOOP('',(#7605,#7606,#7607,#7608));
#2932=EDGE_LOOP('',(#7609,#7610,#7611,#7612));
#2933=EDGE_LOOP('',(#7613,#7614,#7615,#7616));
#2934=EDGE_LOOP('',(#7617,#7618,#7619,#7620));
#2935=EDGE_LOOP('',(#7621,#7622,#7623,#7624));
#2936=EDGE_LOOP('',(#7625,#7626,#7627,#7628));
#2937=EDGE_LOOP('',(#7629,#7630,#7631,#7632));
#2938=EDGE_LOOP('',(#7633,#7634,#7635,#7636));
#2939=EDGE_LOOP('',(#7637,#7638,#7639,#7640));
#2940=EDGE_LOOP('',(#7641,#7642,#7643,#7644));
#2941=EDGE_LOOP('',(#7645,#7646,#7647,#7648));
#2942=EDGE_LOOP('',(#7649,#7650,#7651,#7652));
#2943=EDGE_LOOP('',(#7653,#7654,#7655,#7656));
#2944=EDGE_LOOP('',(#7657,#7658,#7659,#7660));
#2945=EDGE_LOOP('',(#7661,#7662,#7663,#7664));
#2946=EDGE_LOOP('',(#7665,#7666,#7667,#7668));
#2947=EDGE_LOOP('',(#7669,#7670,#7671,#7672));
#2948=EDGE_LOOP('',(#7673,#7674,#7675,#7676));
#2949=EDGE_LOOP('',(#7677,#7678,#7679,#7680));
#2950=EDGE_LOOP('',(#7681,#7682,#7683,#7684));
#2951=EDGE_LOOP('',(#7685,#7686,#7687,#7688));
#2952=EDGE_LOOP('',(#7689,#7690,#7691,#7692));
#2953=EDGE_LOOP('',(#7693,#7694,#7695,#7696));
#2954=EDGE_LOOP('',(#7697,#7698,#7699,#7700));
#2955=EDGE_LOOP('',(#7701,#7702,#7703,#7704));
#2956=EDGE_LOOP('',(#7705,#7706,#7707,#7708,#7709));
#2957=EDGE_LOOP('',(#7710,#7711,#7712,#7713));
#2958=EDGE_LOOP('',(#7714,#7715,#7716,#7717));
#2959=EDGE_LOOP('',(#7718,#7719,#7720,#7721));
#2960=EDGE_LOOP('',(#7722,#7723,#7724,#7725));
#2961=EDGE_LOOP('',(#7726,#7727,#7728,#7729));
#2962=EDGE_LOOP('',(#7730,#7731,#7732,#7733));
#2963=EDGE_LOOP('',(#7734,#7735,#7736,#7737,#7738));
#2964=EDGE_LOOP('',(#7739,#7740,#7741,#7742));
#2965=EDGE_LOOP('',(#7743,#7744,#7745,#7746));
#2966=EDGE_LOOP('',(#7747,#7748,#7749,#7750));
#2967=EDGE_LOOP('',(#7751,#7752,#7753,#7754));
#2968=EDGE_LOOP('',(#7755,#7756,#7757,#7758));
#2969=EDGE_LOOP('',(#7759,#7760,#7761));
#2970=EDGE_LOOP('',(#7762,#7763,#7764,#7765));
#2971=EDGE_LOOP('',(#7766,#7767,#7768));
#2972=EDGE_LOOP('',(#7769,#7770,#7771,#7772));
#2973=EDGE_LOOP('',(#7773,#7774,#7775,#7776));
#2974=EDGE_LOOP('',(#7777,#7778,#7779,#7780));
#2975=EDGE_LOOP('',(#7781,#7782,#7783,#7784));
#2976=EDGE_LOOP('',(#7785,#7786,#7787,#7788));
#3314=CIRCLE('',#9517,5.9);
#3315=CIRCLE('',#9518,0.500000000000001);
#3316=CIRCLE('',#9519,6.4);
#3317=CIRCLE('',#9520,0.500000000000001);
#3318=CIRCLE('',#9522,6.4);
#3319=CIRCLE('',#9523,0.500000000000001);
#3320=CIRCLE('',#9524,5.9);
#3321=CIRCLE('',#9525,0.500000000000001);
#3322=CIRCLE('',#9527,1.5);
#3323=CIRCLE('',#9528,1.5);
#3324=CIRCLE('',#9530,2.00000000000001);
#3325=CIRCLE('',#9531,2.00000000000001);
#3326=CIRCLE('',#9533,2.);
#3327=CIRCLE('',#9534,2.);
#3328=CIRCLE('',#9536,14.1232719083235);
#3329=CIRCLE('',#9537,1.);
#3330=CIRCLE('',#9538,14.989297312108);
#3331=CIRCLE('',#9540,14.989297312108);
#3332=CIRCLE('',#9541,1.);
#3333=CIRCLE('',#9542,14.1232719083235);
#3334=CIRCLE('',#9544,100.);
#3335=CIRCLE('',#9545,100.);
#3336=CIRCLE('',#9548,100.);
#3337=CIRCLE('',#9549,100.);
#3338=CIRCLE('',#9551,100.);
#3339=CIRCLE('',#9552,390.917804157437);
#3340=CIRCLE('',#9553,100.);
#3341=CIRCLE('',#9554,100.);
#3342=CIRCLE('',#9555,390.917804135939);
#3343=CIRCLE('',#9556,100.);
#3344=CIRCLE('',#9558,100.);
#3345=CIRCLE('',#9559,100.);
#3346=CIRCLE('',#9561,3.);
#3347=CIRCLE('',#9562,3.);
#3348=CIRCLE('',#9564,12.5);
#3349=CIRCLE('',#9565,100.5);
#3350=CIRCLE('',#9566,6.44337567297407);
#3351=CIRCLE('',#9567,106.443375672974);
#3352=CIRCLE('',#9568,27.5);
#3353=CIRCLE('',#9569,35.5);
#3354=CIRCLE('',#9570,3.5);
#3355=CIRCLE('',#9571,15.5);
#3356=CIRCLE('',#9572,6.50000000000001);
#3357=CIRCLE('',#9574,12.5);
#3358=CIRCLE('',#9575,6.50000000000001);
#3359=CIRCLE('',#9576,15.5);
#3360=CIRCLE('',#9577,3.5);
#3361=CIRCLE('',#9578,35.5);
#3362=CIRCLE('',#9579,27.5);
#3363=CIRCLE('',#9580,106.443375672974);
#3364=CIRCLE('',#9581,6.44337567297407);
#3365=CIRCLE('',#9582,100.5);
#3366=CIRCLE('',#9585,16.);
#3367=CIRCLE('',#9586,16.);
#3368=CIRCLE('',#9587,16.);
#3369=CIRCLE('',#9588,16.);
#3370=CIRCLE('',#9590,7.);
#3371=CIRCLE('',#9591,7.);
#3372=CIRCLE('',#9593,12.);
#3373=CIRCLE('',#9594,12.);
#3374=CIRCLE('',#9598,28.);
#3375=CIRCLE('',#9599,28.);
#3376=CIRCLE('',#9602,35.);
#3377=CIRCLE('',#9603,35.);
#3378=CIRCLE('',#9605,5.);
#3379=CIRCLE('',#9606,105.);
#3380=CIRCLE('',#9607,13.5459216391339);
#3381=CIRCLE('',#9609,105.57735026919);
#3382=CIRCLE('',#9613,601.835963345588);
#3383=CIRCLE('',#9614,5.57735026918963);
#3384=CIRCLE('',#9616,5.57735026918963);
#3385=CIRCLE('',#9617,601.835963357857);
#3386=CIRCLE('',#9618,5.);
#3387=CIRCLE('',#9621,13.5459216391339);
#3388=CIRCLE('',#9623,105.57735026919);
#3389=CIRCLE('',#9624,105.);
#3390=CIRCLE('',#9627,0.999999999999998);
#3391=CIRCLE('',#9630,0.999999999999998);
#3392=CIRCLE('',#9633,3.);
#3393=CIRCLE('',#9634,3.);
#3394=CIRCLE('',#9637,3.7);
#3395=CIRCLE('',#9639,3.7);
#3396=CIRCLE('',#9661,0.5);
#3397=CIRCLE('',#9662,0.500000000000001);
#3398=CIRCLE('',#9664,0.500000000000001);
#3399=CIRCLE('',#9667,0.500000000000003);
#3400=CIRCLE('',#9669,0.499999999999998);
#3401=CIRCLE('',#9670,0.500000000000005);
#3402=CIRCLE('',#9672,0.5);
#3403=CIRCLE('',#9673,0.500000000000001);
#3404=CIRCLE('',#9675,0.500000000000001);
#3405=CIRCLE('',#9678,0.500000000000003);
#3406=CIRCLE('',#9680,0.499999999999998);
#3407=CIRCLE('',#9681,0.499999999999992);
#3408=CIRCLE('',#9682,0.500000000000009);
#3409=CIRCLE('',#9683,0.499999999999998);
#3410=CIRCLE('',#9685,0.499999999999998);
#3411=CIRCLE('',#9687,0.5);
#3412=CIRCLE('',#9689,0.5);
#3413=CIRCLE('',#9691,0.499999999999999);
#3414=CIRCLE('',#9693,0.499999999999999);
#3415=CIRCLE('',#9695,0.5);
#3416=CIRCLE('',#9697,0.5);
#3417=CIRCLE('',#9699,0.499999999999998);
#3418=CIRCLE('',#9701,0.499999999999998);
#3419=CIRCLE('',#9702,0.500000000000009);
#4059=VERTEX_POINT('',#44356);
#4060=VERTEX_POINT('',#44357);
#4061=VERTEX_POINT('',#44359);
#4062=VERTEX_POINT('',#44361);
#4063=VERTEX_POINT('',#44365);
#4064=VERTEX_POINT('',#44366);
#4065=VERTEX_POINT('',#44368);
#4066=VERTEX_POINT('',#44370);
#4067=VERTEX_POINT('',#44374);
#4068=VERTEX_POINT('',#44376);
#4069=VERTEX_POINT('',#44380);
#4070=VERTEX_POINT('',#44382);
#4071=VERTEX_POINT('',#44386);
#4072=VERTEX_POINT('',#44388);
#4073=VERTEX_POINT('',#44392);
#4074=VERTEX_POINT('',#44393);
#4075=VERTEX_POINT('',#44395);
#4076=VERTEX_POINT('',#44397);
#4077=VERTEX_POINT('',#44443);
#4078=VERTEX_POINT('',#44444);
#4079=VERTEX_POINT('',#44446);
#4080=VERTEX_POINT('',#44448);
#4081=VERTEX_POINT('',#44459);
#4082=VERTEX_POINT('',#44460);
#4083=VERTEX_POINT('',#44462);
#4084=VERTEX_POINT('',#44464);
#4085=VERTEX_POINT('',#44471);
#4086=VERTEX_POINT('',#44472);
#4087=VERTEX_POINT('',#44474);
#4088=VERTEX_POINT('',#44476);
#4089=VERTEX_POINT('',#44480);
#4090=VERTEX_POINT('',#44481);
#4091=VERTEX_POINT('',#44483);
#4092=VERTEX_POINT('',#44485);
#4093=VERTEX_POINT('',#44526);
#4094=VERTEX_POINT('',#44528);
#4095=VERTEX_POINT('',#44530);
#4096=VERTEX_POINT('',#44532);
#4097=VERTEX_POINT('',#44570);
#4098=VERTEX_POINT('',#44572);
#4099=VERTEX_POINT('',#44576);
#4100=VERTEX_POINT('',#44577);
#4101=VERTEX_POINT('',#44579);
#4102=VERTEX_POINT('',#44581);
#4103=VERTEX_POINT('',#44585);
#4104=VERTEX_POINT('',#44586);
#4105=VERTEX_POINT('',#44588);
#4106=VERTEX_POINT('',#44590);
#4107=VERTEX_POINT('',#44594);
#4108=VERTEX_POINT('',#44595);
#4109=VERTEX_POINT('',#44597);
#4110=VERTEX_POINT('',#44599);
#4111=VERTEX_POINT('',#44602);
#4112=VERTEX_POINT('',#44605);
#4113=VERTEX_POINT('',#44607);
#4114=VERTEX_POINT('',#44609);
#4115=VERTEX_POINT('',#44613);
#4116=VERTEX_POINT('',#44614);
#4117=VERTEX_POINT('',#44616);
#4118=VERTEX_POINT('',#44618);
#4119=VERTEX_POINT('',#44620);
#4120=VERTEX_POINT('',#44623);
#4121=VERTEX_POINT('',#44626);
#4122=VERTEX_POINT('',#44628);
#4123=VERTEX_POINT('',#44633);
#4124=VERTEX_POINT('',#44635);
#4125=VERTEX_POINT('',#44637);
#4126=VERTEX_POINT('',#44639);
#4127=VERTEX_POINT('',#44643);
#4128=VERTEX_POINT('',#44645);
#4129=VERTEX_POINT('',#44647);
#4130=VERTEX_POINT('',#44649);
#4131=VERTEX_POINT('',#44651);
#4132=VERTEX_POINT('',#44653);
#4133=VERTEX_POINT('',#44657);
#4134=VERTEX_POINT('',#44658);
#4135=VERTEX_POINT('',#44660);
#4136=VERTEX_POINT('',#44662);
#4137=VERTEX_POINT('',#44669);
#4138=VERTEX_POINT('',#44671);
#4139=VERTEX_POINT('',#44675);
#4140=VERTEX_POINT('',#44677);
#4141=VERTEX_POINT('',#44685);
#4142=VERTEX_POINT('',#44717);
#4143=VERTEX_POINT('',#44719);
#4144=VERTEX_POINT('',#44721);
#4145=VERTEX_POINT('',#44723);
#4146=VERTEX_POINT('',#44752);
#4147=VERTEX_POINT('',#44765);
#4148=VERTEX_POINT('',#44778);
#4149=VERTEX_POINT('',#44780);
#4150=VERTEX_POINT('',#44782);
#4151=VERTEX_POINT('',#44784);
#4152=VERTEX_POINT('',#44792);
#4153=VERTEX_POINT('',#44794);
#4154=VERTEX_POINT('',#44796);
#4155=VERTEX_POINT('',#44798);
#4156=VERTEX_POINT('',#44800);
#4157=VERTEX_POINT('',#44802);
#4158=VERTEX_POINT('',#44804);
#4159=VERTEX_POINT('',#44806);
#4160=VERTEX_POINT('',#44808);
#4161=VERTEX_POINT('',#44810);
#4162=VERTEX_POINT('',#44812);
#4163=VERTEX_POINT('',#44814);
#4164=VERTEX_POINT('',#44816);
#4165=VERTEX_POINT('',#44819);
#4166=VERTEX_POINT('',#44822);
#4167=VERTEX_POINT('',#44826);
#4168=VERTEX_POINT('',#44843);
#4169=VERTEX_POINT('',#44847);
#4170=VERTEX_POINT('',#44848);
#4171=VERTEX_POINT('',#44850);
#4172=VERTEX_POINT('',#44852);
#4173=VERTEX_POINT('',#44856);
#4174=VERTEX_POINT('',#44865);
#4175=VERTEX_POINT('',#44866);
#4176=VERTEX_POINT('',#44889);
#4177=VERTEX_POINT('',#44892);
#4178=VERTEX_POINT('',#44895);
#4179=VERTEX_POINT('',#44897);
#4180=VERTEX_POINT('',#44899);
#4181=VERTEX_POINT('',#44901);
#4182=VERTEX_POINT('',#44903);
#4183=VERTEX_POINT('',#44905);
#4184=VERTEX_POINT('',#44907);
#4185=VERTEX_POINT('',#44909);
#4186=VERTEX_POINT('',#44911);
#4187=VERTEX_POINT('',#44913);
#4188=VERTEX_POINT('',#44915);
#4189=VERTEX_POINT('',#44917);
#4190=VERTEX_POINT('',#44919);
#4191=VERTEX_POINT('',#45009);
#4192=VERTEX_POINT('',#45011);
#4193=VERTEX_POINT('',#45015);
#4194=VERTEX_POINT('',#45019);
#5199=EDGE_CURVE('',#4059,#4060,#3314,.T.);
#5200=EDGE_CURVE('',#4061,#4059,#3315,.T.);
#5201=EDGE_CURVE('',#4062,#4061,#3316,.T.);
#5202=EDGE_CURVE('',#4062,#4060,#3317,.T.);
#5203=EDGE_CURVE('',#4063,#4064,#3318,.T.);
#5204=EDGE_CURVE('',#4065,#4063,#3319,.T.);
#5205=EDGE_CURVE('',#4066,#4065,#3320,.T.);
#5206=EDGE_CURVE('',#4066,#4064,#3321,.T.);
#5207=EDGE_CURVE('',#4067,#4067,#3322,.T.);
#5208=EDGE_CURVE('',#4067,#4068,#1146,.T.);
#5209=EDGE_CURVE('',#4068,#4068,#3323,.T.);
#5210=EDGE_CURVE('',#4069,#4069,#3324,.T.);
#5211=EDGE_CURVE('',#4069,#4070,#1147,.T.);
#5212=EDGE_CURVE('',#4070,#4070,#3325,.T.);
#5213=EDGE_CURVE('',#4071,#4071,#3326,.T.);
#5214=EDGE_CURVE('',#4071,#4072,#1148,.T.);
#5215=EDGE_CURVE('',#4072,#4072,#3327,.T.);
#5216=EDGE_CURVE('',#4073,#4074,#3328,.T.);
#5217=EDGE_CURVE('',#4073,#4075,#3329,.T.);
#5218=EDGE_CURVE('',#4076,#4075,#3330,.T.);
#5219=EDGE_CURVE('',#4076,#4074,#453,.T.);
#5220=EDGE_CURVE('',#4077,#4078,#3331,.T.);
#5221=EDGE_CURVE('',#4077,#4079,#3332,.T.);
#5222=EDGE_CURVE('',#4080,#4079,#3333,.T.);
#5223=EDGE_CURVE('',#4080,#4078,#454,.T.);
#5224=EDGE_CURVE('',#4081,#4082,#3334,.T.);
#5225=EDGE_CURVE('',#4081,#4083,#1149,.T.);
#5226=EDGE_CURVE('',#4083,#4084,#3335,.T.);
#5227=EDGE_CURVE('',#4082,#4084,#1150,.T.);
#5228=EDGE_CURVE('',#4061,#4063,#1151,.T.);
#5229=EDGE_CURVE('',#4062,#4064,#1152,.T.);
#5230=EDGE_CURVE('',#4085,#4086,#3336,.T.);
#5231=EDGE_CURVE('',#4086,#4087,#1153,.T.);
#5232=EDGE_CURVE('',#4088,#4087,#3337,.T.);
#5233=EDGE_CURVE('',#4088,#4085,#1154,.T.);
#5234=EDGE_CURVE('',#4089,#4090,#3338,.T.);
#5235=EDGE_CURVE('',#4089,#4091,#3339,.T.);
#5236=EDGE_CURVE('',#4091,#4092,#455,.T.);
#5237=EDGE_CURVE('',#4092,#4093,#3340,.T.);
#5238=EDGE_CURVE('',#4093,#4094,#1155,.T.);
#5239=EDGE_CURVE('',#4094,#4095,#3341,.T.);
#5240=EDGE_CURVE('',#4095,#4096,#456,.T.);
#5241=EDGE_CURVE('',#4096,#4097,#3342,.T.);
#5242=EDGE_CURVE('',#4097,#4098,#3343,.T.);
#5243=EDGE_CURVE('',#4098,#4090,#1156,.T.);
#5244=EDGE_CURVE('',#4099,#4100,#3344,.T.);
#5245=EDGE_CURVE('',#4100,#4101,#1157,.T.);
#5246=EDGE_CURVE('',#4102,#4101,#3345,.T.);
#5247=EDGE_CURVE('',#4102,#4099,#1158,.T.);
#5248=EDGE_CURVE('',#4103,#4104,#1159,.T.);
#5249=EDGE_CURVE('',#4103,#4105,#3346,.T.);
#5250=EDGE_CURVE('',#4106,#4105,#1160,.T.);
#5251=EDGE_CURVE('',#4104,#4106,#3347,.T.);
#5252=EDGE_CURVE('',#4107,#4108,#3348,.T.);
#5253=EDGE_CURVE('',#4108,#4109,#3349,.T.);
#5254=EDGE_CURVE('',#4109,#4110,#3350,.T.);
#5255=EDGE_CURVE('',#4110,#4077,#3351,.T.);
#5256=EDGE_CURVE('',#4078,#4111,#3352,.T.);
#5257=EDGE_CURVE('',#4111,#4059,#3353,.T.);
#5258=EDGE_CURVE('',#4060,#4112,#1161,.T.);
#5259=EDGE_CURVE('',#4112,#4113,#3354,.T.);
#5260=EDGE_CURVE('',#4113,#4114,#3355,.T.);
#5261=EDGE_CURVE('',#4114,#4107,#3356,.T.);
#5262=EDGE_CURVE('',#4115,#4116,#3357,.T.);
#5263=EDGE_CURVE('',#4116,#4117,#3358,.T.);
#5264=EDGE_CURVE('',#4117,#4118,#3359,.T.);
#5265=EDGE_CURVE('',#4118,#4119,#3360,.T.);
#5266=EDGE_CURVE('',#4119,#4066,#1162,.T.);
#5267=EDGE_CURVE('',#4065,#4120,#3361,.T.);
#5268=EDGE_CURVE('',#4120,#4076,#3362,.T.);
#5269=EDGE_CURVE('',#4075,#4121,#3363,.T.);
#5270=EDGE_CURVE('',#4121,#4122,#3364,.T.);
#5271=EDGE_CURVE('',#4122,#4115,#3365,.T.);
#5272=EDGE_CURVE('',#4064,#4103,#1163,.T.);
#5273=EDGE_CURVE('',#4104,#4123,#1164,.T.);
#5274=EDGE_CURVE('',#4124,#4123,#1165,.T.);
#5275=EDGE_CURVE('',#4125,#4124,#1166,.T.);
#5276=EDGE_CURVE('',#4125,#4126,#1167,.T.);
#5277=EDGE_CURVE('',#4126,#4062,#1168,.T.);
#5278=EDGE_CURVE('',#4105,#4127,#3366,.T.);
#5279=EDGE_CURVE('',#4127,#4128,#1169,.T.);
#5280=EDGE_CURVE('',#4128,#4129,#3367,.T.);
#5281=EDGE_CURVE('',#4129,#4130,#1170,.T.);
#5282=EDGE_CURVE('',#4130,#4131,#3368,.T.);
#5283=EDGE_CURVE('',#4132,#4131,#1171,.T.);
#5284=EDGE_CURVE('',#4106,#4132,#3369,.T.);
#5285=EDGE_CURVE('',#4133,#4134,#1172,.T.);
#5286=EDGE_CURVE('',#4133,#4135,#3370,.T.);
#5287=EDGE_CURVE('',#4135,#4136,#1173,.T.);
#5288=EDGE_CURVE('',#4136,#4134,#3371,.T.);
#5289=EDGE_CURVE('',#4093,#4133,#3372,.T.);
#5290=EDGE_CURVE('',#4134,#4094,#3373,.T.);
#5291=EDGE_CURVE('',#4084,#4137,#1174,.T.);
#5292=EDGE_CURVE('',#4138,#4137,#1175,.T.);
#5293=EDGE_CURVE('',#4082,#4138,#1176,.T.);
#5294=EDGE_CURVE('',#4137,#4139,#111,.T.);
#5295=EDGE_CURVE('',#4139,#4140,#457,.T.);
#5296=EDGE_CURVE('',#4140,#4141,#458,.T.);
#5297=EDGE_CURVE('',#4141,#4142,#3374,.T.);
#5298=EDGE_CURVE('',#4143,#4142,#1177,.T.);
#5299=EDGE_CURVE('',#4143,#4144,#3375,.T.);
#5300=EDGE_CURVE('',#4144,#4145,#459,.T.);
#5301=EDGE_CURVE('',#4145,#4146,#460,.T.);
#5302=EDGE_CURVE('',#4138,#4146,#112,.T.);
#5303=EDGE_CURVE('',#4061,#4143,#3376,.T.);
#5304=EDGE_CURVE('',#4142,#4063,#3377,.T.);
#5305=EDGE_CURVE('',#4097,#4147,#461,.T.);
#5306=EDGE_CURVE('',#4147,#4148,#3378,.T.);
#5307=EDGE_CURVE('',#4149,#4148,#3379,.T.);
#5308=EDGE_CURVE('',#4150,#4149,#3380,.T.);
#5309=EDGE_CURVE('',#4150,#4151,#462,.T.);
#5310=EDGE_CURVE('',#4137,#4151,#1178,.T.);
#5311=EDGE_CURVE('',#4083,#4152,#1179,.T.);
#5312=EDGE_CURVE('',#4152,#4153,#1180,.T.);
#5313=EDGE_CURVE('',#4153,#4154,#1181,.T.);
#5314=EDGE_CURVE('',#4154,#4155,#1182,.T.);
#5315=EDGE_CURVE('',#4155,#4156,#1183,.T.);
#5316=EDGE_CURVE('',#4156,#4157,#1184,.T.);
#5317=EDGE_CURVE('',#4157,#4158,#1185,.T.);
#5318=EDGE_CURVE('',#4158,#4159,#1186,.T.);
#5319=EDGE_CURVE('',#4159,#4160,#1187,.T.);
#5320=EDGE_CURVE('',#4160,#4161,#1188,.T.);
#5321=EDGE_CURVE('',#4161,#4162,#1189,.T.);
#5322=EDGE_CURVE('',#4162,#4163,#1190,.T.);
#5323=EDGE_CURVE('',#4163,#4164,#1191,.T.);
#5324=EDGE_CURVE('',#4164,#4100,#1192,.T.);
#5325=EDGE_CURVE('',#4099,#4165,#1193,.T.);
#5326=EDGE_CURVE('',#4165,#4086,#1194,.T.);
#5327=EDGE_CURVE('',#4085,#4166,#1195,.T.);
#5328=EDGE_CURVE('',#4166,#4098,#1196,.T.);
#5329=EDGE_CURVE('',#4167,#4148,#1197,.T.);
#5330=EDGE_CURVE('',#4167,#4073,#3381,.T.);
#5331=EDGE_CURVE('',#4073,#4149,#1198,.T.);
#5332=EDGE_CURVE('',#4074,#4150,#463,.T.);
#5333=EDGE_CURVE('',#4151,#4139,#464,.T.);
#5334=EDGE_CURVE('',#4147,#4168,#3382,.T.);
#5335=EDGE_CURVE('',#4168,#4167,#3383,.T.);
#5336=EDGE_CURVE('',#4169,#4170,#3384,.T.);
#5337=EDGE_CURVE('',#4170,#4171,#3385,.T.);
#5338=EDGE_CURVE('',#4171,#4172,#3386,.T.);
#5339=EDGE_CURVE('',#4172,#4169,#1199,.T.);
#5340=EDGE_CURVE('',#4146,#4173,#465,.T.);
#5341=EDGE_CURVE('',#4138,#4173,#1200,.T.);
#5342=EDGE_CURVE('',#4174,#4175,#3387,.T.);
#5343=EDGE_CURVE('',#4174,#4080,#466,.T.);
#5344=EDGE_CURVE('',#4175,#4079,#1201,.T.);
#5345=EDGE_CURVE('',#4079,#4169,#3388,.T.);
#5346=EDGE_CURVE('',#4175,#4172,#3389,.T.);
#5347=EDGE_CURVE('',#4171,#4089,#467,.T.);
#5348=EDGE_CURVE('',#4176,#4090,#1202,.T.);
#5349=EDGE_CURVE('',#4088,#4176,#1203,.T.);
#5350=EDGE_CURVE('',#4177,#4087,#1204,.T.);
#5351=EDGE_CURVE('',#4102,#4177,#1205,.T.);
#5352=EDGE_CURVE('',#4178,#4101,#1206,.T.);
#5353=EDGE_CURVE('',#4179,#4178,#1207,.T.);
#5354=EDGE_CURVE('',#4180,#4179,#1208,.T.);
#5355=EDGE_CURVE('',#4181,#4180,#1209,.T.);
#5356=EDGE_CURVE('',#4182,#4181,#1210,.T.);
#5357=EDGE_CURVE('',#4183,#4182,#1211,.T.);
#5358=EDGE_CURVE('',#4184,#4183,#1212,.T.);
#5359=EDGE_CURVE('',#4185,#4184,#1213,.T.);
#5360=EDGE_CURVE('',#4186,#4185,#1214,.T.);
#5361=EDGE_CURVE('',#4187,#4186,#1215,.T.);
#5362=EDGE_CURVE('',#4188,#4187,#1216,.T.);
#5363=EDGE_CURVE('',#4189,#4188,#1217,.T.);
#5364=EDGE_CURVE('',#4190,#4189,#1218,.T.);
#5365=EDGE_CURVE('',#4081,#4190,#1219,.T.);
#5366=EDGE_CURVE('',#4173,#4174,#468,.T.);
#5367=EDGE_CURVE('',#4109,#4170,#469,.T.);
#5368=EDGE_CURVE('',#4110,#4169,#3390,.T.);
#5369=EDGE_CURVE('',#4168,#4122,#470,.T.);
#5370=EDGE_CURVE('',#4167,#4121,#3391,.T.);
#5371=EDGE_CURVE('',#4129,#4126,#3392,.T.);
#5372=EDGE_CURVE('',#4125,#4130,#3393,.T.);
#5373=EDGE_CURVE('',#4191,#4132,#1220,.T.);
#5374=EDGE_CURVE('',#4192,#4131,#1221,.T.);
#5375=EDGE_CURVE('',#4192,#4191,#1222,.T.);
#5376=EDGE_CURVE('',#4124,#4193,#1223,.T.);
#5377=EDGE_CURVE('',#4193,#4192,#3394,.T.);
#5378=EDGE_CURVE('',#4194,#4191,#3395,.T.);
#5379=EDGE_CURVE('',#4123,#4194,#1224,.T.);
#5380=EDGE_CURVE('',#4193,#4194,#1225,.T.);
#5381=EDGE_CURVE('',#4189,#4153,#1226,.T.);
#5382=EDGE_CURVE('',#4152,#4190,#1227,.T.);
#5383=EDGE_CURVE('',#4154,#4188,#1228,.T.);
#5384=EDGE_CURVE('',#4156,#4186,#1229,.T.);
#5385=EDGE_CURVE('',#4187,#4155,#1230,.T.);
#5386=EDGE_CURVE('',#4158,#4184,#1231,.T.);
#5387=EDGE_CURVE('',#4185,#4157,#1232,.T.);
#5388=EDGE_CURVE('',#4160,#4182,#1233,.T.);
#5389=EDGE_CURVE('',#4183,#4159,#1234,.T.);
#5390=EDGE_CURVE('',#4162,#4180,#1235,.T.);
#5391=EDGE_CURVE('',#4181,#4161,#1236,.T.);
#5392=EDGE_CURVE('',#4164,#4178,#1237,.T.);
#5393=EDGE_CURVE('',#4179,#4163,#1238,.T.);
#5394=EDGE_CURVE('',#4166,#4176,#1239,.T.);
#5395=EDGE_CURVE('',#4165,#4177,#1240,.T.);
#5396=EDGE_CURVE('',#4117,#4127,#3396,.T.);
#5397=EDGE_CURVE('',#4118,#4105,#3397,.T.);
#5398=EDGE_CURVE('',#4119,#4103,#3398,.T.);
#5399=EDGE_CURVE('',#4120,#4142,#3399,.T.);
#5400=EDGE_CURVE('',#4076,#4141,#3400,.T.);
#5401=EDGE_CURVE('',#4074,#4140,#3401,.T.);
#5402=EDGE_CURVE('',#4128,#4114,#3402,.T.);
#5403=EDGE_CURVE('',#4129,#4113,#3403,.T.);
#5404=EDGE_CURVE('',#4126,#4112,#3404,.T.);
#5405=EDGE_CURVE('',#4143,#4111,#3405,.T.);
#5406=EDGE_CURVE('',#4144,#4078,#3406,.T.);
#5407=EDGE_CURVE('',#4145,#4080,#3407,.T.);
#5408=EDGE_CURVE('',#4168,#4096,#3408,.T.);
#5409=EDGE_CURVE('',#4122,#4095,#3409,.T.);
#5410=EDGE_CURVE('',#4115,#4094,#3410,.T.);
#5411=EDGE_CURVE('',#4116,#4134,#3411,.T.);
#5412=EDGE_CURVE('',#4117,#4136,#3412,.T.);
#5413=EDGE_CURVE('',#4127,#4136,#3413,.T.);
#5414=EDGE_CURVE('',#4128,#4135,#3414,.T.);
#5415=EDGE_CURVE('',#4114,#4135,#3415,.T.);
#5416=EDGE_CURVE('',#4107,#4133,#3416,.T.);
#5417=EDGE_CURVE('',#4108,#4093,#3417,.T.);
#5418=EDGE_CURVE('',#4109,#4092,#3418,.T.);
#5419=EDGE_CURVE('',#4170,#4091,#3419,.T.);
#7347=ORIENTED_EDGE('',*,*,#5199,.F.);
#7348=ORIENTED_EDGE('',*,*,#5200,.F.);
#7349=ORIENTED_EDGE('',*,*,#5201,.F.);
#7350=ORIENTED_EDGE('',*,*,#5202,.T.);
#7351=ORIENTED_EDGE('',*,*,#5203,.F.);
#7352=ORIENTED_EDGE('',*,*,#5204,.F.);
#7353=ORIENTED_EDGE('',*,*,#5205,.F.);
#7354=ORIENTED_EDGE('',*,*,#5206,.T.);
#7355=ORIENTED_EDGE('',*,*,#5207,.T.);
#7356=ORIENTED_EDGE('',*,*,#5208,.T.);
#7357=ORIENTED_EDGE('',*,*,#5209,.F.);
#7358=ORIENTED_EDGE('',*,*,#5208,.F.);
#7359=ORIENTED_EDGE('',*,*,#5210,.T.);
#7360=ORIENTED_EDGE('',*,*,#5211,.T.);
#7361=ORIENTED_EDGE('',*,*,#5212,.T.);
#7362=ORIENTED_EDGE('',*,*,#5211,.F.);
#7363=ORIENTED_EDGE('',*,*,#5213,.T.);
#7364=ORIENTED_EDGE('',*,*,#5214,.T.);
#7365=ORIENTED_EDGE('',*,*,#5215,.T.);
#7366=ORIENTED_EDGE('',*,*,#5214,.F.);
#7367=ORIENTED_EDGE('',*,*,#5216,.F.);
#7368=ORIENTED_EDGE('',*,*,#5217,.T.);
#7369=ORIENTED_EDGE('',*,*,#5218,.F.);
#7370=ORIENTED_EDGE('',*,*,#5219,.T.);
#7371=ORIENTED_EDGE('',*,*,#5220,.F.);
#7372=ORIENTED_EDGE('',*,*,#5221,.T.);
#7373=ORIENTED_EDGE('',*,*,#5222,.F.);
#7374=ORIENTED_EDGE('',*,*,#5223,.T.);
#7375=ORIENTED_EDGE('',*,*,#5224,.F.);
#7376=ORIENTED_EDGE('',*,*,#5225,.T.);
#7377=ORIENTED_EDGE('',*,*,#5226,.T.);
#7378=ORIENTED_EDGE('',*,*,#5227,.F.);
#7379=ORIENTED_EDGE('',*,*,#5201,.T.);
#7380=ORIENTED_EDGE('',*,*,#5228,.T.);
#7381=ORIENTED_EDGE('',*,*,#5203,.T.);
#7382=ORIENTED_EDGE('',*,*,#5229,.F.);
#7383=ORIENTED_EDGE('',*,*,#5230,.T.);
#7384=ORIENTED_EDGE('',*,*,#5231,.T.);
#7385=ORIENTED_EDGE('',*,*,#5232,.F.);
#7386=ORIENTED_EDGE('',*,*,#5233,.T.);
#7387=ORIENTED_EDGE('',*,*,#5234,.F.);
#7388=ORIENTED_EDGE('',*,*,#5235,.T.);
#7389=ORIENTED_EDGE('',*,*,#5236,.T.);
#7390=ORIENTED_EDGE('',*,*,#5237,.T.);
#7391=ORIENTED_EDGE('',*,*,#5238,.T.);
#7392=ORIENTED_EDGE('',*,*,#5239,.T.);
#7393=ORIENTED_EDGE('',*,*,#5240,.T.);
#7394=ORIENTED_EDGE('',*,*,#5241,.T.);
#7395=ORIENTED_EDGE('',*,*,#5242,.T.);
#7396=ORIENTED_EDGE('',*,*,#5243,.T.);
#7397=ORIENTED_EDGE('',*,*,#5244,.T.);
#7398=ORIENTED_EDGE('',*,*,#5245,.T.);
#7399=ORIENTED_EDGE('',*,*,#5246,.F.);
#7400=ORIENTED_EDGE('',*,*,#5247,.T.);
#7401=ORIENTED_EDGE('',*,*,#5248,.F.);
#7402=ORIENTED_EDGE('',*,*,#5249,.T.);
#7403=ORIENTED_EDGE('',*,*,#5250,.F.);
#7404=ORIENTED_EDGE('',*,*,#5251,.F.);
#7405=ORIENTED_EDGE('',*,*,#5252,.T.);
#7406=ORIENTED_EDGE('',*,*,#5253,.T.);
#7407=ORIENTED_EDGE('',*,*,#5254,.T.);
#7408=ORIENTED_EDGE('',*,*,#5255,.T.);
#7409=ORIENTED_EDGE('',*,*,#5220,.T.);
#7410=ORIENTED_EDGE('',*,*,#5256,.T.);
#7411=ORIENTED_EDGE('',*,*,#5257,.T.);
#7412=ORIENTED_EDGE('',*,*,#5199,.T.);
#7413=ORIENTED_EDGE('',*,*,#5258,.T.);
#7414=ORIENTED_EDGE('',*,*,#5259,.T.);
#7415=ORIENTED_EDGE('',*,*,#5260,.T.);
#7416=ORIENTED_EDGE('',*,*,#5261,.T.);
#7417=ORIENTED_EDGE('',*,*,#5212,.F.);
#7418=ORIENTED_EDGE('',*,*,#5215,.F.);
#7419=ORIENTED_EDGE('',*,*,#5262,.T.);
#7420=ORIENTED_EDGE('',*,*,#5263,.T.);
#7421=ORIENTED_EDGE('',*,*,#5264,.T.);
#7422=ORIENTED_EDGE('',*,*,#5265,.T.);
#7423=ORIENTED_EDGE('',*,*,#5266,.T.);
#7424=ORIENTED_EDGE('',*,*,#5205,.T.);
#7425=ORIENTED_EDGE('',*,*,#5267,.T.);
#7426=ORIENTED_EDGE('',*,*,#5268,.T.);
#7427=ORIENTED_EDGE('',*,*,#5218,.T.);
#7428=ORIENTED_EDGE('',*,*,#5269,.T.);
#7429=ORIENTED_EDGE('',*,*,#5270,.T.);
#7430=ORIENTED_EDGE('',*,*,#5271,.T.);
#7431=ORIENTED_EDGE('',*,*,#5210,.F.);
#7432=ORIENTED_EDGE('',*,*,#5213,.F.);
#7433=ORIENTED_EDGE('',*,*,#5229,.T.);
#7434=ORIENTED_EDGE('',*,*,#5272,.T.);
#7435=ORIENTED_EDGE('',*,*,#5248,.T.);
#7436=ORIENTED_EDGE('',*,*,#5273,.T.);
#7437=ORIENTED_EDGE('',*,*,#5274,.F.);
#7438=ORIENTED_EDGE('',*,*,#5275,.F.);
#7439=ORIENTED_EDGE('',*,*,#5276,.T.);
#7440=ORIENTED_EDGE('',*,*,#5277,.T.);
#7441=ORIENTED_EDGE('',*,*,#5278,.T.);
#7442=ORIENTED_EDGE('',*,*,#5279,.T.);
#7443=ORIENTED_EDGE('',*,*,#5280,.T.);
#7444=ORIENTED_EDGE('',*,*,#5281,.T.);
#7445=ORIENTED_EDGE('',*,*,#5282,.T.);
#7446=ORIENTED_EDGE('',*,*,#5283,.F.);
#7447=ORIENTED_EDGE('',*,*,#5284,.F.);
#7448=ORIENTED_EDGE('',*,*,#5250,.T.);
#7449=ORIENTED_EDGE('',*,*,#5285,.F.);
#7450=ORIENTED_EDGE('',*,*,#5286,.T.);
#7451=ORIENTED_EDGE('',*,*,#5287,.T.);
#7452=ORIENTED_EDGE('',*,*,#5288,.T.);
#7453=ORIENTED_EDGE('',*,*,#5238,.F.);
#7454=ORIENTED_EDGE('',*,*,#5289,.T.);
#7455=ORIENTED_EDGE('',*,*,#5285,.T.);
#7456=ORIENTED_EDGE('',*,*,#5290,.T.);
#7457=ORIENTED_EDGE('',*,*,#5227,.T.);
#7458=ORIENTED_EDGE('',*,*,#5291,.T.);
#7459=ORIENTED_EDGE('',*,*,#5292,.F.);
#7460=ORIENTED_EDGE('',*,*,#5293,.F.);
#7461=ORIENTED_EDGE('',*,*,#5294,.T.);
#7462=ORIENTED_EDGE('',*,*,#5295,.T.);
#7463=ORIENTED_EDGE('',*,*,#5296,.T.);
#7464=ORIENTED_EDGE('',*,*,#5297,.T.);
#7465=ORIENTED_EDGE('',*,*,#5298,.F.);
#7466=ORIENTED_EDGE('',*,*,#5299,.T.);
#7467=ORIENTED_EDGE('',*,*,#5300,.T.);
#7468=ORIENTED_EDGE('',*,*,#5301,.T.);
#7469=ORIENTED_EDGE('',*,*,#5302,.F.);
#7470=ORIENTED_EDGE('',*,*,#5292,.T.);
#7471=ORIENTED_EDGE('',*,*,#5228,.F.);
#7472=ORIENTED_EDGE('',*,*,#5303,.T.);
#7473=ORIENTED_EDGE('',*,*,#5298,.T.);
#7474=ORIENTED_EDGE('',*,*,#5304,.T.);
#7475=ORIENTED_EDGE('',*,*,#5242,.F.);
#7476=ORIENTED_EDGE('',*,*,#5305,.T.);
#7477=ORIENTED_EDGE('',*,*,#5306,.T.);
#7478=ORIENTED_EDGE('',*,*,#5307,.F.);
#7479=ORIENTED_EDGE('',*,*,#5308,.F.);
#7480=ORIENTED_EDGE('',*,*,#5309,.T.);
#7481=ORIENTED_EDGE('',*,*,#5310,.F.);
#7482=ORIENTED_EDGE('',*,*,#5291,.F.);
#7483=ORIENTED_EDGE('',*,*,#5226,.F.);
#7484=ORIENTED_EDGE('',*,*,#5311,.T.);
#7485=ORIENTED_EDGE('',*,*,#5312,.T.);
#7486=ORIENTED_EDGE('',*,*,#5313,.T.);
#7487=ORIENTED_EDGE('',*,*,#5314,.T.);
#7488=ORIENTED_EDGE('',*,*,#5315,.T.);
#7489=ORIENTED_EDGE('',*,*,#5316,.T.);
#7490=ORIENTED_EDGE('',*,*,#5317,.T.);
#7491=ORIENTED_EDGE('',*,*,#5318,.T.);
#7492=ORIENTED_EDGE('',*,*,#5319,.T.);
#7493=ORIENTED_EDGE('',*,*,#5320,.T.);
#7494=ORIENTED_EDGE('',*,*,#5321,.T.);
#7495=ORIENTED_EDGE('',*,*,#5322,.T.);
#7496=ORIENTED_EDGE('',*,*,#5323,.T.);
#7497=ORIENTED_EDGE('',*,*,#5324,.T.);
#7498=ORIENTED_EDGE('',*,*,#5244,.F.);
#7499=ORIENTED_EDGE('',*,*,#5325,.T.);
#7500=ORIENTED_EDGE('',*,*,#5326,.T.);
#7501=ORIENTED_EDGE('',*,*,#5230,.F.);
#7502=ORIENTED_EDGE('',*,*,#5327,.T.);
#7503=ORIENTED_EDGE('',*,*,#5328,.T.);
#7504=ORIENTED_EDGE('',*,*,#5329,.F.);
#7505=ORIENTED_EDGE('',*,*,#5330,.T.);
#7506=ORIENTED_EDGE('',*,*,#5331,.T.);
#7507=ORIENTED_EDGE('',*,*,#5307,.T.);
#7508=ORIENTED_EDGE('',*,*,#5216,.T.);
#7509=ORIENTED_EDGE('',*,*,#5332,.T.);
#7510=ORIENTED_EDGE('',*,*,#5308,.T.);
#7511=ORIENTED_EDGE('',*,*,#5331,.F.);
#7512=ORIENTED_EDGE('',*,*,#5310,.T.);
#7513=ORIENTED_EDGE('',*,*,#5333,.T.);
#7514=ORIENTED_EDGE('',*,*,#5294,.F.);
#7515=ORIENTED_EDGE('',*,*,#5306,.F.);
#7516=ORIENTED_EDGE('',*,*,#5334,.T.);
#7517=ORIENTED_EDGE('',*,*,#5335,.T.);
#7518=ORIENTED_EDGE('',*,*,#5329,.T.);
#7519=ORIENTED_EDGE('',*,*,#5336,.T.);
#7520=ORIENTED_EDGE('',*,*,#5337,.T.);
#7521=ORIENTED_EDGE('',*,*,#5338,.T.);
#7522=ORIENTED_EDGE('',*,*,#5339,.T.);
#7523=ORIENTED_EDGE('',*,*,#5302,.T.);
#7524=ORIENTED_EDGE('',*,*,#5340,.T.);
#7525=ORIENTED_EDGE('',*,*,#5341,.F.);
#7526=ORIENTED_EDGE('',*,*,#5342,.F.);
#7527=ORIENTED_EDGE('',*,*,#5343,.T.);
#7528=ORIENTED_EDGE('',*,*,#5222,.T.);
#7529=ORIENTED_EDGE('',*,*,#5344,.F.);
#7530=ORIENTED_EDGE('',*,*,#5344,.T.);
#7531=ORIENTED_EDGE('',*,*,#5345,.T.);
#7532=ORIENTED_EDGE('',*,*,#5339,.F.);
#7533=ORIENTED_EDGE('',*,*,#5346,.F.);
#7534=ORIENTED_EDGE('',*,*,#5338,.F.);
#7535=ORIENTED_EDGE('',*,*,#5347,.T.);
#7536=ORIENTED_EDGE('',*,*,#5234,.T.);
#7537=ORIENTED_EDGE('',*,*,#5348,.F.);
#7538=ORIENTED_EDGE('',*,*,#5349,.F.);
#7539=ORIENTED_EDGE('',*,*,#5232,.T.);
#7540=ORIENTED_EDGE('',*,*,#5350,.F.);
#7541=ORIENTED_EDGE('',*,*,#5351,.F.);
#7542=ORIENTED_EDGE('',*,*,#5246,.T.);
#7543=ORIENTED_EDGE('',*,*,#5352,.F.);
#7544=ORIENTED_EDGE('',*,*,#5353,.F.);
#7545=ORIENTED_EDGE('',*,*,#5354,.F.);
#7546=ORIENTED_EDGE('',*,*,#5355,.F.);
#7547=ORIENTED_EDGE('',*,*,#5356,.F.);
#7548=ORIENTED_EDGE('',*,*,#5357,.F.);
#7549=ORIENTED_EDGE('',*,*,#5358,.F.);
#7550=ORIENTED_EDGE('',*,*,#5359,.F.);
#7551=ORIENTED_EDGE('',*,*,#5360,.F.);
#7552=ORIENTED_EDGE('',*,*,#5361,.F.);
#7553=ORIENTED_EDGE('',*,*,#5362,.F.);
#7554=ORIENTED_EDGE('',*,*,#5363,.F.);
#7555=ORIENTED_EDGE('',*,*,#5364,.F.);
#7556=ORIENTED_EDGE('',*,*,#5365,.F.);
#7557=ORIENTED_EDGE('',*,*,#5224,.T.);
#7558=ORIENTED_EDGE('',*,*,#5293,.T.);
#7559=ORIENTED_EDGE('',*,*,#5341,.T.);
#7560=ORIENTED_EDGE('',*,*,#5366,.T.);
#7561=ORIENTED_EDGE('',*,*,#5342,.T.);
#7562=ORIENTED_EDGE('',*,*,#5346,.T.);
#7563=ORIENTED_EDGE('',*,*,#5254,.F.);
#7564=ORIENTED_EDGE('',*,*,#5367,.T.);
#7565=ORIENTED_EDGE('',*,*,#5336,.F.);
#7566=ORIENTED_EDGE('',*,*,#5368,.F.);
#7567=ORIENTED_EDGE('',*,*,#5368,.T.);
#7568=ORIENTED_EDGE('',*,*,#5345,.F.);
#7569=ORIENTED_EDGE('',*,*,#5221,.F.);
#7570=ORIENTED_EDGE('',*,*,#5255,.F.);
#7571=ORIENTED_EDGE('',*,*,#5335,.F.);
#7572=ORIENTED_EDGE('',*,*,#5369,.T.);
#7573=ORIENTED_EDGE('',*,*,#5270,.F.);
#7574=ORIENTED_EDGE('',*,*,#5370,.F.);
#7575=ORIENTED_EDGE('',*,*,#5370,.T.);
#7576=ORIENTED_EDGE('',*,*,#5269,.F.);
#7577=ORIENTED_EDGE('',*,*,#5217,.F.);
#7578=ORIENTED_EDGE('',*,*,#5330,.F.);
#7579=ORIENTED_EDGE('',*,*,#5281,.F.);
#7580=ORIENTED_EDGE('',*,*,#5371,.T.);
#7581=ORIENTED_EDGE('',*,*,#5276,.F.);
#7582=ORIENTED_EDGE('',*,*,#5372,.T.);
#7583=ORIENTED_EDGE('',*,*,#5373,.T.);
#7584=ORIENTED_EDGE('',*,*,#5283,.T.);
#7585=ORIENTED_EDGE('',*,*,#5374,.F.);
#7586=ORIENTED_EDGE('',*,*,#5375,.T.);
#7587=ORIENTED_EDGE('',*,*,#5282,.F.);
#7588=ORIENTED_EDGE('',*,*,#5372,.F.);
#7589=ORIENTED_EDGE('',*,*,#5275,.T.);
#7590=ORIENTED_EDGE('',*,*,#5376,.T.);
#7591=ORIENTED_EDGE('',*,*,#5377,.T.);
#7592=ORIENTED_EDGE('',*,*,#5374,.T.);
#7593=ORIENTED_EDGE('',*,*,#5207,.F.);
#7594=ORIENTED_EDGE('',*,*,#5251,.T.);
#7595=ORIENTED_EDGE('',*,*,#5284,.T.);
#7596=ORIENTED_EDGE('',*,*,#5373,.F.);
#7597=ORIENTED_EDGE('',*,*,#5378,.F.);
#7598=ORIENTED_EDGE('',*,*,#5379,.F.);
#7599=ORIENTED_EDGE('',*,*,#5273,.F.);
#7600=ORIENTED_EDGE('',*,*,#5209,.T.);
#7601=ORIENTED_EDGE('',*,*,#5378,.T.);
#7602=ORIENTED_EDGE('',*,*,#5375,.F.);
#7603=ORIENTED_EDGE('',*,*,#5377,.F.);
#7604=ORIENTED_EDGE('',*,*,#5380,.T.);
#7605=ORIENTED_EDGE('',*,*,#5379,.T.);
#7606=ORIENTED_EDGE('',*,*,#5380,.F.);
#7607=ORIENTED_EDGE('',*,*,#5376,.F.);
#7608=ORIENTED_EDGE('',*,*,#5274,.T.);
#7609=ORIENTED_EDGE('',*,*,#5364,.T.);
#7610=ORIENTED_EDGE('',*,*,#5381,.T.);
#7611=ORIENTED_EDGE('',*,*,#5312,.F.);
#7612=ORIENTED_EDGE('',*,*,#5382,.T.);
#7613=ORIENTED_EDGE('',*,*,#5365,.T.);
#7614=ORIENTED_EDGE('',*,*,#5382,.F.);
#7615=ORIENTED_EDGE('',*,*,#5311,.F.);
#7616=ORIENTED_EDGE('',*,*,#5225,.F.);
#7617=ORIENTED_EDGE('',*,*,#5363,.T.);
#7618=ORIENTED_EDGE('',*,*,#5383,.F.);
#7619=ORIENTED_EDGE('',*,*,#5313,.F.);
#7620=ORIENTED_EDGE('',*,*,#5381,.F.);
#7621=ORIENTED_EDGE('',*,*,#5361,.T.);
#7622=ORIENTED_EDGE('',*,*,#5384,.F.);
#7623=ORIENTED_EDGE('',*,*,#5315,.F.);
#7624=ORIENTED_EDGE('',*,*,#5385,.F.);
#7625=ORIENTED_EDGE('',*,*,#5359,.T.);
#7626=ORIENTED_EDGE('',*,*,#5386,.F.);
#7627=ORIENTED_EDGE('',*,*,#5317,.F.);
#7628=ORIENTED_EDGE('',*,*,#5387,.F.);
#7629=ORIENTED_EDGE('',*,*,#5357,.T.);
#7630=ORIENTED_EDGE('',*,*,#5388,.F.);
#7631=ORIENTED_EDGE('',*,*,#5319,.F.);
#7632=ORIENTED_EDGE('',*,*,#5389,.F.);
#7633=ORIENTED_EDGE('',*,*,#5355,.T.);
#7634=ORIENTED_EDGE('',*,*,#5390,.F.);
#7635=ORIENTED_EDGE('',*,*,#5321,.F.);
#7636=ORIENTED_EDGE('',*,*,#5391,.F.);
#7637=ORIENTED_EDGE('',*,*,#5353,.T.);
#7638=ORIENTED_EDGE('',*,*,#5392,.F.);
#7639=ORIENTED_EDGE('',*,*,#5323,.F.);
#7640=ORIENTED_EDGE('',*,*,#5393,.F.);
#7641=ORIENTED_EDGE('',*,*,#5324,.F.);
#7642=ORIENTED_EDGE('',*,*,#5392,.T.);
#7643=ORIENTED_EDGE('',*,*,#5352,.T.);
#7644=ORIENTED_EDGE('',*,*,#5245,.F.);
#7645=ORIENTED_EDGE('',*,*,#5393,.T.);
#7646=ORIENTED_EDGE('',*,*,#5322,.F.);
#7647=ORIENTED_EDGE('',*,*,#5390,.T.);
#7648=ORIENTED_EDGE('',*,*,#5354,.T.);
#7649=ORIENTED_EDGE('',*,*,#5391,.T.);
#7650=ORIENTED_EDGE('',*,*,#5320,.F.);
#7651=ORIENTED_EDGE('',*,*,#5388,.T.);
#7652=ORIENTED_EDGE('',*,*,#5356,.T.);
#7653=ORIENTED_EDGE('',*,*,#5389,.T.);
#7654=ORIENTED_EDGE('',*,*,#5318,.F.);
#7655=ORIENTED_EDGE('',*,*,#5386,.T.);
#7656=ORIENTED_EDGE('',*,*,#5358,.T.);
#7657=ORIENTED_EDGE('',*,*,#5387,.T.);
#7658=ORIENTED_EDGE('',*,*,#5316,.F.);
#7659=ORIENTED_EDGE('',*,*,#5384,.T.);
#7660=ORIENTED_EDGE('',*,*,#5360,.T.);
#7661=ORIENTED_EDGE('',*,*,#5385,.T.);
#7662=ORIENTED_EDGE('',*,*,#5314,.F.);
#7663=ORIENTED_EDGE('',*,*,#5383,.T.);
#7664=ORIENTED_EDGE('',*,*,#5362,.T.);
#7665=ORIENTED_EDGE('',*,*,#5349,.T.);
#7666=ORIENTED_EDGE('',*,*,#5394,.F.);
#7667=ORIENTED_EDGE('',*,*,#5327,.F.);
#7668=ORIENTED_EDGE('',*,*,#5233,.F.);
#7669=ORIENTED_EDGE('',*,*,#5328,.F.);
#7670=ORIENTED_EDGE('',*,*,#5394,.T.);
#7671=ORIENTED_EDGE('',*,*,#5348,.T.);
#7672=ORIENTED_EDGE('',*,*,#5243,.F.);
#7673=ORIENTED_EDGE('',*,*,#5326,.F.);
#7674=ORIENTED_EDGE('',*,*,#5395,.T.);
#7675=ORIENTED_EDGE('',*,*,#5350,.T.);
#7676=ORIENTED_EDGE('',*,*,#5231,.F.);
#7677=ORIENTED_EDGE('',*,*,#5351,.T.);
#7678=ORIENTED_EDGE('',*,*,#5395,.F.);
#7679=ORIENTED_EDGE('',*,*,#5325,.F.);
#7680=ORIENTED_EDGE('',*,*,#5247,.F.);
#7681=ORIENTED_EDGE('',*,*,#5264,.F.);
#7682=ORIENTED_EDGE('',*,*,#5396,.T.);
#7683=ORIENTED_EDGE('',*,*,#5278,.F.);
#7684=ORIENTED_EDGE('',*,*,#5397,.F.);
#7685=ORIENTED_EDGE('',*,*,#5397,.T.);
#7686=ORIENTED_EDGE('',*,*,#5249,.F.);
#7687=ORIENTED_EDGE('',*,*,#5398,.F.);
#7688=ORIENTED_EDGE('',*,*,#5265,.F.);
#7689=ORIENTED_EDGE('',*,*,#5398,.T.);
#7690=ORIENTED_EDGE('',*,*,#5272,.F.);
#7691=ORIENTED_EDGE('',*,*,#5206,.F.);
#7692=ORIENTED_EDGE('',*,*,#5266,.F.);
#7693=ORIENTED_EDGE('',*,*,#5204,.T.);
#7694=ORIENTED_EDGE('',*,*,#5304,.F.);
#7695=ORIENTED_EDGE('',*,*,#5399,.F.);
#7696=ORIENTED_EDGE('',*,*,#5267,.F.);
#7697=ORIENTED_EDGE('',*,*,#5399,.T.);
#7698=ORIENTED_EDGE('',*,*,#5297,.F.);
#7699=ORIENTED_EDGE('',*,*,#5400,.F.);
#7700=ORIENTED_EDGE('',*,*,#5268,.F.);
#7701=ORIENTED_EDGE('',*,*,#5400,.T.);
#7702=ORIENTED_EDGE('',*,*,#5296,.F.);
#7703=ORIENTED_EDGE('',*,*,#5401,.F.);
#7704=ORIENTED_EDGE('',*,*,#5219,.F.);
#7705=ORIENTED_EDGE('',*,*,#5309,.F.);
#7706=ORIENTED_EDGE('',*,*,#5332,.F.);
#7707=ORIENTED_EDGE('',*,*,#5401,.T.);
#7708=ORIENTED_EDGE('',*,*,#5295,.F.);
#7709=ORIENTED_EDGE('',*,*,#5333,.F.);
#7710=ORIENTED_EDGE('',*,*,#5280,.F.);
#7711=ORIENTED_EDGE('',*,*,#5402,.T.);
#7712=ORIENTED_EDGE('',*,*,#5260,.F.);
#7713=ORIENTED_EDGE('',*,*,#5403,.F.);
#7714=ORIENTED_EDGE('',*,*,#5403,.T.);
#7715=ORIENTED_EDGE('',*,*,#5259,.F.);
#7716=ORIENTED_EDGE('',*,*,#5404,.F.);
#7717=ORIENTED_EDGE('',*,*,#5371,.F.);
#7718=ORIENTED_EDGE('',*,*,#5404,.T.);
#7719=ORIENTED_EDGE('',*,*,#5258,.F.);
#7720=ORIENTED_EDGE('',*,*,#5202,.F.);
#7721=ORIENTED_EDGE('',*,*,#5277,.F.);
#7722=ORIENTED_EDGE('',*,*,#5200,.T.);
#7723=ORIENTED_EDGE('',*,*,#5257,.F.);
#7724=ORIENTED_EDGE('',*,*,#5405,.F.);
#7725=ORIENTED_EDGE('',*,*,#5303,.F.);
#7726=ORIENTED_EDGE('',*,*,#5405,.T.);
#7727=ORIENTED_EDGE('',*,*,#5256,.F.);
#7728=ORIENTED_EDGE('',*,*,#5406,.F.);
#7729=ORIENTED_EDGE('',*,*,#5299,.F.);
#7730=ORIENTED_EDGE('',*,*,#5406,.T.);
#7731=ORIENTED_EDGE('',*,*,#5223,.F.);
#7732=ORIENTED_EDGE('',*,*,#5407,.F.);
#7733=ORIENTED_EDGE('',*,*,#5300,.F.);
#7734=ORIENTED_EDGE('',*,*,#5340,.F.);
#7735=ORIENTED_EDGE('',*,*,#5301,.F.);
#7736=ORIENTED_EDGE('',*,*,#5407,.T.);
#7737=ORIENTED_EDGE('',*,*,#5343,.F.);
#7738=ORIENTED_EDGE('',*,*,#5366,.F.);
#7739=ORIENTED_EDGE('',*,*,#5305,.F.);
#7740=ORIENTED_EDGE('',*,*,#5241,.F.);
#7741=ORIENTED_EDGE('',*,*,#5408,.F.);
#7742=ORIENTED_EDGE('',*,*,#5334,.F.);
#7743=ORIENTED_EDGE('',*,*,#5408,.T.);
#7744=ORIENTED_EDGE('',*,*,#5240,.F.);
#7745=ORIENTED_EDGE('',*,*,#5409,.F.);
#7746=ORIENTED_EDGE('',*,*,#5369,.F.);
#7747=ORIENTED_EDGE('',*,*,#5409,.T.);
#7748=ORIENTED_EDGE('',*,*,#5239,.F.);
#7749=ORIENTED_EDGE('',*,*,#5410,.F.);
#7750=ORIENTED_EDGE('',*,*,#5271,.F.);
#7751=ORIENTED_EDGE('',*,*,#5410,.T.);
#7752=ORIENTED_EDGE('',*,*,#5290,.F.);
#7753=ORIENTED_EDGE('',*,*,#5411,.F.);
#7754=ORIENTED_EDGE('',*,*,#5262,.F.);
#7755=ORIENTED_EDGE('',*,*,#5412,.F.);
#7756=ORIENTED_EDGE('',*,*,#5263,.F.);
#7757=ORIENTED_EDGE('',*,*,#5411,.T.);
#7758=ORIENTED_EDGE('',*,*,#5288,.F.);
#7759=ORIENTED_EDGE('',*,*,#5396,.F.);
#7760=ORIENTED_EDGE('',*,*,#5412,.T.);
#7761=ORIENTED_EDGE('',*,*,#5413,.F.);
#7762=ORIENTED_EDGE('',*,*,#5414,.F.);
#7763=ORIENTED_EDGE('',*,*,#5279,.F.);
#7764=ORIENTED_EDGE('',*,*,#5413,.T.);
#7765=ORIENTED_EDGE('',*,*,#5287,.F.);
#7766=ORIENTED_EDGE('',*,*,#5402,.F.);
#7767=ORIENTED_EDGE('',*,*,#5414,.T.);
#7768=ORIENTED_EDGE('',*,*,#5415,.F.);
#7769=ORIENTED_EDGE('',*,*,#5415,.T.);
#7770=ORIENTED_EDGE('',*,*,#5286,.F.);
#7771=ORIENTED_EDGE('',*,*,#5416,.F.);
#7772=ORIENTED_EDGE('',*,*,#5261,.F.);
#7773=ORIENTED_EDGE('',*,*,#5416,.T.);
#7774=ORIENTED_EDGE('',*,*,#5289,.F.);
#7775=ORIENTED_EDGE('',*,*,#5417,.F.);
#7776=ORIENTED_EDGE('',*,*,#5252,.F.);
#7777=ORIENTED_EDGE('',*,*,#5417,.T.);
#7778=ORIENTED_EDGE('',*,*,#5237,.F.);
#7779=ORIENTED_EDGE('',*,*,#5418,.F.);
#7780=ORIENTED_EDGE('',*,*,#5253,.F.);
#7781=ORIENTED_EDGE('',*,*,#5418,.T.);
#7782=ORIENTED_EDGE('',*,*,#5236,.F.);
#7783=ORIENTED_EDGE('',*,*,#5419,.F.);
#7784=ORIENTED_EDGE('',*,*,#5367,.F.);
#7785=ORIENTED_EDGE('',*,*,#5347,.F.);
#7786=ORIENTED_EDGE('',*,*,#5337,.F.);
#7787=ORIENTED_EDGE('',*,*,#5419,.T.);
#7788=ORIENTED_EDGE('',*,*,#5235,.F.);
#8407=SPHERICAL_SURFACE('',#9690,0.5);
#8408=SPHERICAL_SURFACE('',#9694,0.5);
#8713=ADVANCED_FACE('',(#2363),#630,.T.);
#8714=ADVANCED_FACE('',(#2364),#631,.T.);
#8715=ADVANCED_FACE('',(#2365),#1998,.F.);
#8716=ADVANCED_FACE('',(#2366),#1999,.F.);
#8717=ADVANCED_FACE('',(#2367),#2000,.F.);
#8718=ADVANCED_FACE('',(#2368),#632,.F.);
#8719=ADVANCED_FACE('',(#2369),#633,.F.);
#8720=ADVANCED_FACE('',(#2370),#2001,.F.);
#8721=ADVANCED_FACE('',(#2371),#2002,.T.);
#8722=ADVANCED_FACE('',(#2372),#2003,.F.);
#8723=ADVANCED_FACE('',(#2373),#2004,.F.);
#8724=ADVANCED_FACE('',(#2374),#2005,.F.);
#8725=ADVANCED_FACE('',(#2375),#2006,.F.);
#8726=ADVANCED_FACE('',(#2376,#731,#732),#812,.F.);
#8727=ADVANCED_FACE('',(#2377,#733,#734),#813,.T.);
#8728=ADVANCED_FACE('',(#2378),#814,.F.);
#8729=ADVANCED_FACE('',(#2379),#2007,.T.);
#8730=ADVANCED_FACE('',(#2380),#2008,.T.);
#8731=ADVANCED_FACE('',(#2381),#2009,.F.);
#8732=ADVANCED_FACE('',(#2382),#815,.F.);
#8733=ADVANCED_FACE('',(#2383),#2010,.T.);
#8734=ADVANCED_FACE('',(#2384),#2011,.F.);
#8735=ADVANCED_FACE('',(#2385),#816,.F.);
#8736=ADVANCED_FACE('',(#2386),#142,.T.);
#8737=ADVANCED_FACE('',(#2387),#143,.T.);
#8738=ADVANCED_FACE('',(#2388),#817,.T.);
#8739=ADVANCED_FACE('',(#2389),#144,.T.);
#8740=ADVANCED_FACE('',(#2390),#145,.T.);
#8741=ADVANCED_FACE('',(#2391),#818,.T.);
#8742=ADVANCED_FACE('',(#2392),#146,.T.);
#8743=ADVANCED_FACE('',(#2393),#147,.T.);
#8744=ADVANCED_FACE('',(#2394),#819,.T.);
#8745=ADVANCED_FACE('',(#2395),#634,.F.);
#8746=ADVANCED_FACE('',(#2396),#635,.F.);
#8747=ADVANCED_FACE('',(#2397),#636,.F.);
#8748=ADVANCED_FACE('',(#2398),#637,.F.);
#8749=ADVANCED_FACE('',(#2399),#2012,.F.);
#8750=ADVANCED_FACE('',(#2400),#820,.F.);
#8751=ADVANCED_FACE('',(#2401,#735),#821,.T.);
#8752=ADVANCED_FACE('',(#2402,#736),#822,.F.);
#8753=ADVANCED_FACE('',(#2403),#2013,.T.);
#8754=ADVANCED_FACE('',(#2404),#823,.F.);
#8755=ADVANCED_FACE('',(#2405),#824,.F.);
#8756=ADVANCED_FACE('',(#2406),#825,.F.);
#8757=ADVANCED_FACE('',(#2407),#826,.F.);
#8758=ADVANCED_FACE('',(#2408),#827,.F.);
#8759=ADVANCED_FACE('',(#2409),#828,.F.);
#8760=ADVANCED_FACE('',(#2410),#829,.F.);
#8761=ADVANCED_FACE('',(#2411),#830,.F.);
#8762=ADVANCED_FACE('',(#2412),#831,.F.);
#8763=ADVANCED_FACE('',(#2413),#832,.F.);
#8764=ADVANCED_FACE('',(#2414),#833,.F.);
#8765=ADVANCED_FACE('',(#2415),#834,.F.);
#8766=ADVANCED_FACE('',(#2416),#835,.F.);
#8767=ADVANCED_FACE('',(#2417),#836,.F.);
#8768=ADVANCED_FACE('',(#2418),#837,.F.);
#8769=ADVANCED_FACE('',(#2419),#838,.F.);
#8770=ADVANCED_FACE('',(#2420),#839,.F.);
#8771=ADVANCED_FACE('',(#2421),#840,.F.);
#8772=ADVANCED_FACE('',(#2422),#841,.F.);
#8773=ADVANCED_FACE('',(#2423),#638,.T.);
#8774=ADVANCED_FACE('',(#2424),#639,.T.);
#8775=ADVANCED_FACE('',(#2425),#2014,.T.);
#8776=ADVANCED_FACE('',(#2426),#640,.T.);
#8777=ADVANCED_FACE('',(#2427),#641,.T.);
#8778=ADVANCED_FACE('',(#2428),#590,.T.);
#8779=ADVANCED_FACE('',(#2429),#591,.T.);
#8780=ADVANCED_FACE('',(#2430),#642,.T.);
#8781=ADVANCED_FACE('',(#2431),#643,.T.);
#8782=ADVANCED_FACE('',(#2432),#2015,.T.);
#8783=ADVANCED_FACE('',(#2433),#644,.T.);
#8784=ADVANCED_FACE('',(#2434),#645,.T.);
#8785=ADVANCED_FACE('',(#2435),#592,.T.);
#8786=ADVANCED_FACE('',(#2436),#593,.T.);
#8787=ADVANCED_FACE('',(#2437),#594,.T.);
#8788=ADVANCED_FACE('',(#2438),#595,.T.);
#8789=ADVANCED_FACE('',(#2439),#646,.T.);
#8790=ADVANCED_FACE('',(#2440),#647,.T.);
#8791=ADVANCED_FACE('',(#2441),#648,.T.);
#8792=ADVANCED_FACE('',(#2442),#8407,.T.);
#8793=ADVANCED_FACE('',(#2443),#2016,.T.);
#8794=ADVANCED_FACE('',(#2444),#8408,.T.);
#8795=ADVANCED_FACE('',(#2445),#649,.T.);
#8796=ADVANCED_FACE('',(#2446),#650,.T.);
#8797=ADVANCED_FACE('',(#2447),#651,.T.);
#8798=ADVANCED_FACE('',(#2448),#596,.T.);
#8799=ADVANCED_FACE('',(#2449),#597,.T.);
#8931=CLOSED_SHELL('',(#8713,#8714,#8715,#8716,#8717,#8718,#8719,#8720,
#8721,#8722,#8723,#8724,#8725,#8726,#8727,#8728,#8729,#8730,#8731,#8732,
#8733,#8734,#8735,#8736,#8737,#8738,#8739,#8740,#8741,#8742,#8743,#8744,
#8745,#8746,#8747,#8748,#8749,#8750,#8751,#8752,#8753,#8754,#8755,#8756,
#8757,#8758,#8759,#8760,#8761,#8762,#8763,#8764,#8765,#8766,#8767,#8768,
#8769,#8770,#8771,#8772,#8773,#8774,#8775,#8776,#8777,#8778,#8779,#8780,
#8781,#8782,#8783,#8784,#8785,#8786,#8787,#8788,#8789,#8790,#8791,#8792,
#8793,#8794,#8795,#8796,#8797,#8798,#8799));
#9515=AXIS2_PLACEMENT_3D('',#44354,#11109,#11110);
#9516=AXIS2_PLACEMENT_3D('',#44355,#11111,#11112);
#9517=AXIS2_PLACEMENT_3D('',#44358,#11113,#11114);
#9518=AXIS2_PLACEMENT_3D('',#44360,#11115,#11116);
#9519=AXIS2_PLACEMENT_3D('',#44362,#11117,#11118);
#9520=AXIS2_PLACEMENT_3D('',#44363,#11119,#11120);
#9521=AXIS2_PLACEMENT_3D('',#44364,#11121,#11122);
#9522=AXIS2_PLACEMENT_3D('',#44367,#11123,#11124);
#9523=AXIS2_PLACEMENT_3D('',#44369,#11125,#11126);
#9524=AXIS2_PLACEMENT_3D('',#44371,#11127,#11128);
#9525=AXIS2_PLACEMENT_3D('',#44372,#11129,#11130);
#9526=AXIS2_PLACEMENT_3D('',#44373,#11131,#11132);
#9527=AXIS2_PLACEMENT_3D('',#44375,#11133,#11134);
#9528=AXIS2_PLACEMENT_3D('',#44378,#11136,#11137);
#9529=AXIS2_PLACEMENT_3D('',#44379,#11138,#11139);
#9530=AXIS2_PLACEMENT_3D('',#44381,#11140,#11141);
#9531=AXIS2_PLACEMENT_3D('',#44384,#11143,#11144);
#9532=AXIS2_PLACEMENT_3D('',#44385,#11145,#11146);
#9533=AXIS2_PLACEMENT_3D('',#44387,#11147,#11148);
#9534=AXIS2_PLACEMENT_3D('',#44390,#11150,#11151);
#9535=AXIS2_PLACEMENT_3D('',#44391,#11152,#11153);
#9536=AXIS2_PLACEMENT_3D('',#44394,#11154,#11155);
#9537=AXIS2_PLACEMENT_3D('',#44396,#11156,#11157);
#9538=AXIS2_PLACEMENT_3D('',#44398,#11158,#11159);
#9539=AXIS2_PLACEMENT_3D('',#44442,#11160,#11161);
#9540=AXIS2_PLACEMENT_3D('',#44445,#11162,#11163);
#9541=AXIS2_PLACEMENT_3D('',#44447,#11164,#11165);
#9542=AXIS2_PLACEMENT_3D('',#44449,#11166,#11167);
#9543=AXIS2_PLACEMENT_3D('',#44458,#11168,#11169);
#9544=AXIS2_PLACEMENT_3D('',#44461,#11170,#11171);
#9545=AXIS2_PLACEMENT_3D('',#44465,#11173,#11174);
#9546=AXIS2_PLACEMENT_3D('',#44467,#11176,#11177);
#9547=AXIS2_PLACEMENT_3D('',#44470,#11180,#11181);
#9548=AXIS2_PLACEMENT_3D('',#44473,#11182,#11183);
#9549=AXIS2_PLACEMENT_3D('',#44477,#11185,#11186);
#9550=AXIS2_PLACEMENT_3D('',#44479,#11188,#11189);
#9551=AXIS2_PLACEMENT_3D('',#44482,#11190,#11191);
#9552=AXIS2_PLACEMENT_3D('',#44484,#11192,#11193);
#9553=AXIS2_PLACEMENT_3D('',#44527,#11194,#11195);
#9554=AXIS2_PLACEMENT_3D('',#44531,#11197,#11198);
#9555=AXIS2_PLACEMENT_3D('',#44571,#11199,#11200);
#9556=AXIS2_PLACEMENT_3D('',#44573,#11201,#11202);
#9557=AXIS2_PLACEMENT_3D('',#44575,#11204,#11205);
#9558=AXIS2_PLACEMENT_3D('',#44578,#11206,#11207);
#9559=AXIS2_PLACEMENT_3D('',#44582,#11209,#11210);
#9560=AXIS2_PLACEMENT_3D('',#44584,#11212,#11213);
#9561=AXIS2_PLACEMENT_3D('',#44589,#11215,#11216);
#9562=AXIS2_PLACEMENT_3D('',#44592,#11218,#11219);
#9563=AXIS2_PLACEMENT_3D('',#44593,#11220,#11221);
#9564=AXIS2_PLACEMENT_3D('',#44596,#11222,#11223);
#9565=AXIS2_PLACEMENT_3D('',#44598,#11224,#11225);
#9566=AXIS2_PLACEMENT_3D('',#44600,#11226,#11227);
#9567=AXIS2_PLACEMENT_3D('',#44601,#11228,#11229);
#9568=AXIS2_PLACEMENT_3D('',#44603,#11230,#11231);
#9569=AXIS2_PLACEMENT_3D('',#44604,#11232,#11233);
#9570=AXIS2_PLACEMENT_3D('',#44608,#11235,#11236);
#9571=AXIS2_PLACEMENT_3D('',#44610,#11237,#11238);
#9572=AXIS2_PLACEMENT_3D('',#44611,#11239,#11240);
#9573=AXIS2_PLACEMENT_3D('',#44612,#11241,#11242);
#9574=AXIS2_PLACEMENT_3D('',#44615,#11243,#11244);
#9575=AXIS2_PLACEMENT_3D('',#44617,#11245,#11246);
#9576=AXIS2_PLACEMENT_3D('',#44619,#11247,#11248);
#9577=AXIS2_PLACEMENT_3D('',#44621,#11249,#11250);
#9578=AXIS2_PLACEMENT_3D('',#44624,#11252,#11253);
#9579=AXIS2_PLACEMENT_3D('',#44625,#11254,#11255);
#9580=AXIS2_PLACEMENT_3D('',#44627,#11256,#11257);
#9581=AXIS2_PLACEMENT_3D('',#44629,#11258,#11259);
#9582=AXIS2_PLACEMENT_3D('',#44630,#11260,#11261);
#9583=AXIS2_PLACEMENT_3D('',#44631,#11262,#11263);
#9584=AXIS2_PLACEMENT_3D('',#44642,#11270,#11271);
#9585=AXIS2_PLACEMENT_3D('',#44644,#11272,#11273);
#9586=AXIS2_PLACEMENT_3D('',#44648,#11275,#11276);
#9587=AXIS2_PLACEMENT_3D('',#44652,#11278,#11279);
#9588=AXIS2_PLACEMENT_3D('',#44655,#11281,#11282);
#9589=AXIS2_PLACEMENT_3D('',#44656,#11283,#11284);
#9590=AXIS2_PLACEMENT_3D('',#44661,#11286,#11287);
#9591=AXIS2_PLACEMENT_3D('',#44664,#11289,#11290);
#9592=AXIS2_PLACEMENT_3D('',#44665,#11291,#11292);
#9593=AXIS2_PLACEMENT_3D('',#44666,#11293,#11294);
#9594=AXIS2_PLACEMENT_3D('',#44667,#11295,#11296);
#9595=AXIS2_PLACEMENT_3D('',#44668,#11297,#11298);
#9596=AXIS2_PLACEMENT_3D('',#44674,#11302,#11303);
#9597=AXIS2_PLACEMENT_3D('',#44676,#11304,#11305);
#9598=AXIS2_PLACEMENT_3D('',#44718,#11306,#11307);
#9599=AXIS2_PLACEMENT_3D('',#44722,#11309,#11310);
#9600=AXIS2_PLACEMENT_3D('',#44760,#11311,#11312);
#9601=AXIS2_PLACEMENT_3D('',#44761,#11313,#11314);
#9602=AXIS2_PLACEMENT_3D('',#44762,#11315,#11316);
#9603=AXIS2_PLACEMENT_3D('',#44763,#11317,#11318);
#9604=AXIS2_PLACEMENT_3D('',#44764,#11319,#11320);
#9605=AXIS2_PLACEMENT_3D('',#44779,#11321,#11322);
#9606=AXIS2_PLACEMENT_3D('',#44781,#11323,#11324);
#9607=AXIS2_PLACEMENT_3D('',#44783,#11325,#11326);
#9608=AXIS2_PLACEMENT_3D('',#44825,#11346,#11347);
#9609=AXIS2_PLACEMENT_3D('',#44828,#11349,#11350);
#9610=AXIS2_PLACEMENT_3D('',#44830,#11352,#11353);
#9611=AXIS2_PLACEMENT_3D('',#44835,#11354,#11355);
#9612=AXIS2_PLACEMENT_3D('',#44842,#11356,#11357);
#9613=AXIS2_PLACEMENT_3D('',#44844,#11358,#11359);
#9614=AXIS2_PLACEMENT_3D('',#44845,#11360,#11361);
#9615=AXIS2_PLACEMENT_3D('',#44846,#11362,#11363);
#9616=AXIS2_PLACEMENT_3D('',#44849,#11364,#11365);
#9617=AXIS2_PLACEMENT_3D('',#44851,#11366,#11367);
#9618=AXIS2_PLACEMENT_3D('',#44853,#11368,#11369);
#9619=AXIS2_PLACEMENT_3D('',#44855,#11371,#11372);
#9620=AXIS2_PLACEMENT_3D('',#44864,#11374,#11375);
#9621=AXIS2_PLACEMENT_3D('',#44867,#11376,#11377);
#9622=AXIS2_PLACEMENT_3D('',#44873,#11379,#11380);
#9623=AXIS2_PLACEMENT_3D('',#44874,#11381,#11382);
#9624=AXIS2_PLACEMENT_3D('',#44875,#11383,#11384);
#9625=AXIS2_PLACEMENT_3D('',#44876,#11385,#11386);
#9626=AXIS2_PLACEMENT_3D('',#44928,#11405,#11406);
#9627=AXIS2_PLACEMENT_3D('',#44963,#11407,#11408);
#9628=AXIS2_PLACEMENT_3D('',#44964,#11409,#11410);
#9629=AXIS2_PLACEMENT_3D('',#44965,#11411,#11412);
#9630=AXIS2_PLACEMENT_3D('',#45003,#11413,#11414);
#9631=AXIS2_PLACEMENT_3D('',#45004,#11415,#11416);
#9632=AXIS2_PLACEMENT_3D('',#45005,#11417,#11418);
#9633=AXIS2_PLACEMENT_3D('',#45006,#11419,#11420);
#9634=AXIS2_PLACEMENT_3D('',#45007,#11421,#11422);
#9635=AXIS2_PLACEMENT_3D('',#45008,#11423,#11424);
#9636=AXIS2_PLACEMENT_3D('',#45014,#11428,#11429);
#9637=AXIS2_PLACEMENT_3D('',#45017,#11431,#11432);
#9638=AXIS2_PLACEMENT_3D('',#45018,#11433,#11434);
#9639=AXIS2_PLACEMENT_3D('',#45020,#11435,#11436);
#9640=AXIS2_PLACEMENT_3D('',#45022,#11438,#11439);
#9641=AXIS2_PLACEMENT_3D('',#45024,#11441,#11442);
#9642=AXIS2_PLACEMENT_3D('',#45025,#11443,#11444);
#9643=AXIS2_PLACEMENT_3D('',#45028,#11447,#11448);
#9644=AXIS2_PLACEMENT_3D('',#45029,#11449,#11450);
#9645=AXIS2_PLACEMENT_3D('',#45031,#11452,#11453);
#9646=AXIS2_PLACEMENT_3D('',#45034,#11456,#11457);
#9647=AXIS2_PLACEMENT_3D('',#45037,#11460,#11461);
#9648=AXIS2_PLACEMENT_3D('',#45040,#11464,#11465);
#9649=AXIS2_PLACEMENT_3D('',#45043,#11468,#11469);
#9650=AXIS2_PLACEMENT_3D('',#45046,#11472,#11473);
#9651=AXIS2_PLACEMENT_3D('',#45047,#11474,#11475);
#9652=AXIS2_PLACEMENT_3D('',#45048,#11476,#11477);
#9653=AXIS2_PLACEMENT_3D('',#45049,#11478,#11479);
#9654=AXIS2_PLACEMENT_3D('',#45050,#11480,#11481);
#9655=AXIS2_PLACEMENT_3D('',#45051,#11482,#11483);
#9656=AXIS2_PLACEMENT_3D('',#45052,#11484,#11485);
#9657=AXIS2_PLACEMENT_3D('',#45054,#11487,#11488);
#9658=AXIS2_PLACEMENT_3D('',#45055,#11489,#11490);
#9659=AXIS2_PLACEMENT_3D('',#45057,#11492,#11493);
#9660=AXIS2_PLACEMENT_3D('',#45058,#11494,#11495);
#9661=AXIS2_PLACEMENT_3D('',#45059,#11496,#11497);
#9662=AXIS2_PLACEMENT_3D('',#45060,#11498,#11499);
#9663=AXIS2_PLACEMENT_3D('',#45061,#11500,#11501);
#9664=AXIS2_PLACEMENT_3D('',#45062,#11502,#11503);
#9665=AXIS2_PLACEMENT_3D('',#45063,#11504,#11505);
#9666=AXIS2_PLACEMENT_3D('',#45064,#11506,#11507);
#9667=AXIS2_PLACEMENT_3D('',#45065,#11508,#11509);
#9668=AXIS2_PLACEMENT_3D('',#45066,#11510,#11511);
#9669=AXIS2_PLACEMENT_3D('',#45067,#11512,#11513);
#9670=AXIS2_PLACEMENT_3D('',#45092,#11514,#11515);
#9671=AXIS2_PLACEMENT_3D('',#45105,#11516,#11517);
#9672=AXIS2_PLACEMENT_3D('',#45106,#11518,#11519);
#9673=AXIS2_PLACEMENT_3D('',#45107,#11520,#11521);
#9674=AXIS2_PLACEMENT_3D('',#45108,#11522,#11523);
#9675=AXIS2_PLACEMENT_3D('',#45109,#11524,#11525);
#9676=AXIS2_PLACEMENT_3D('',#45110,#11526,#11527);
#9677=AXIS2_PLACEMENT_3D('',#45111,#11528,#11529);
#9678=AXIS2_PLACEMENT_3D('',#45112,#11530,#11531);
#9679=AXIS2_PLACEMENT_3D('',#45113,#11532,#11533);
#9680=AXIS2_PLACEMENT_3D('',#45114,#11534,#11535);
#9681=AXIS2_PLACEMENT_3D('',#45139,#11536,#11537);
#9682=AXIS2_PLACEMENT_3D('',#45164,#11538,#11539);
#9683=AXIS2_PLACEMENT_3D('',#45189,#11540,#11541);
#9684=AXIS2_PLACEMENT_3D('',#45190,#11542,#11543);
#9685=AXIS2_PLACEMENT_3D('',#45191,#11544,#11545);
#9686=AXIS2_PLACEMENT_3D('',#45192,#11546,#11547);
#9687=AXIS2_PLACEMENT_3D('',#45193,#11548,#11549);
#9688=AXIS2_PLACEMENT_3D('',#45194,#11550,#11551);
#9689=AXIS2_PLACEMENT_3D('',#45195,#11552,#11553);
#9690=AXIS2_PLACEMENT_3D('',#45196,#11554,#11555);
#9691=AXIS2_PLACEMENT_3D('',#45197,#11556,#11557);
#9692=AXIS2_PLACEMENT_3D('',#45198,#11558,#11559);
#9693=AXIS2_PLACEMENT_3D('',#45199,#11560,#11561);
#9694=AXIS2_PLACEMENT_3D('',#45200,#11562,#11563);
#9695=AXIS2_PLACEMENT_3D('',#45201,#11564,#11565);
#9696=AXIS2_PLACEMENT_3D('',#45202,#11566,#11567);
#9697=AXIS2_PLACEMENT_3D('',#45203,#11568,#11569);
#9698=AXIS2_PLACEMENT_3D('',#45204,#11570,#11571);
#9699=AXIS2_PLACEMENT_3D('',#45205,#11572,#11573);
#9700=AXIS2_PLACEMENT_3D('',#45206,#11574,#11575);
#9701=AXIS2_PLACEMENT_3D('',#45207,#11576,#11577);
#9702=AXIS2_PLACEMENT_3D('',#45232,#11578,#11579);
#11109=DIRECTION('axis',(0.,0.,1.));
#11110=DIRECTION('refdir',(1.,0.,0.));
#11111=DIRECTION('center_axis',(-2.46563637061793E-17,-5.67162995353388E-17,
-1.));
#11112=DIRECTION('ref_axis',(-0.99065493718706,0.136392065117079,0.));
#11113=DIRECTION('center_axis',(2.46563637061793E-17,5.67162995353388E-17,
1.));
#11114=DIRECTION('ref_axis',(-0.99065493718706,0.136392065117079,1.66902952191827E-17));
#11115=DIRECTION('center_axis',(0.813167683561177,0.582029482424859,1.13956207311045E-15));
#11116=DIRECTION('ref_axis',(-0.582029482424859,0.813167683561177,2.73196138259506E-30));
#11117=DIRECTION('center_axis',(-2.46563637061793E-17,-5.67162995353388E-17,
-1.));
#11118=DIRECTION('ref_axis',(-0.99065493718706,0.136392065117079,1.66902952191827E-17));
#11119=DIRECTION('center_axis',(-0.916721549040254,-0.399526721916366,4.52626971630092E-17));
#11120=DIRECTION('ref_axis',(0.399526721916366,-0.916721549040254,2.21817733744602E-31));
#11121=DIRECTION('center_axis',(-2.46563637061793E-17,-5.67162995353388E-17,
-1.));
#11122=DIRECTION('ref_axis',(-0.99065493718706,0.136392065117079,0.));
#11123=DIRECTION('center_axis',(2.46563637061793E-17,5.67162995353388E-17,
1.));
#11124=DIRECTION('ref_axis',(-0.99065493718706,0.136392065117079,1.66902952191827E-17));
#11125=DIRECTION('center_axis',(0.813167683561178,0.582029482424858,-5.30603166236022E-17));
#11126=DIRECTION('ref_axis',(-0.582029482424858,0.813167683561178,-1.88716532676391E-31));
#11127=DIRECTION('center_axis',(-2.46563637061793E-17,-5.67162995353388E-17,
-1.));
#11128=DIRECTION('ref_axis',(-0.99065493718706,0.136392065117079,1.66902952191827E-17));
#11129=DIRECTION('center_axis',(-0.916721549040254,-0.399526721916366,4.52626971630092E-17));
#11130=DIRECTION('ref_axis',(0.399526721916366,-0.916721549040254,2.43484877201396E-31));
#11131=DIRECTION('center_axis',(-2.46563637061793E-17,-5.67162995353388E-17,
-1.));
#11132=DIRECTION('ref_axis',(-0.99065493718706,0.136392065117078,1.66902952191827E-17));
#11133=DIRECTION('center_axis',(2.46563637061793E-17,5.67162995353388E-17,
1.));
#11134=DIRECTION('ref_axis',(0.99065493718706,-0.136392065117078,-1.66902952191827E-17));
#11135=DIRECTION('',(-2.46563637061793E-17,-5.67162995353388E-17,-1.));
#11136=DIRECTION('center_axis',(2.46563637061793E-17,5.67162995353388E-17,
1.));
#11137=DIRECTION('ref_axis',(0.99065493718706,-0.136392065117078,-1.66902952191827E-17));
#11138=DIRECTION('center_axis',(2.46563637061793E-17,5.67162995353388E-17,
1.));
#11139=DIRECTION('ref_axis',(0.99065493718706,-0.136392065117079,-1.66902952191827E-17));
#11140=DIRECTION('center_axis',(-2.46563637061793E-17,-5.67162995353388E-17,
-1.));
#11141=DIRECTION('ref_axis',(-0.99065493718706,0.136392065117079,1.66902952191827E-17));
#11142=DIRECTION('',(2.46563637061793E-17,5.67162995353388E-17,1.));
#11143=DIRECTION('center_axis',(2.46563637061793E-17,5.67162995353388E-17,
1.));
#11144=DIRECTION('ref_axis',(0.99065493718706,-0.136392065117079,-1.66902952191827E-17));
#11145=DIRECTION('center_axis',(2.46563637061793E-17,5.67162995353388E-17,
1.));
#11146=DIRECTION('ref_axis',(0.99065493718706,-0.136392065117079,-1.66902952191827E-17));
#11147=DIRECTION('center_axis',(-2.46563637061793E-17,-5.67162995353388E-17,
-1.));
#11148=DIRECTION('ref_axis',(-0.99065493718706,0.136392065117079,1.66902952191827E-17));
#11149=DIRECTION('',(2.46563637061793E-17,5.67162995353388E-17,1.));
#11150=DIRECTION('center_axis',(2.46563637061793E-17,5.67162995353388E-17,
1.));
#11151=DIRECTION('ref_axis',(0.99065493718706,-0.136392065117079,-1.66902952191827E-17));
#11152=DIRECTION('center_axis',(-2.46563637061793E-17,-5.67162995353388E-17,
-1.));
#11153=DIRECTION('ref_axis',(-0.99065493718706,0.136392065117079,0.));
#11154=DIRECTION('center_axis',(-2.46563637061793E-17,-5.67162995353388E-17,
-1.));
#11155=DIRECTION('ref_axis',(-0.99065493718706,0.136392065117079,1.66902952191827E-17));
#11156=DIRECTION('center_axis',(-0.089158316805357,-0.996017466987621,9.09675535379384E-13));
#11157=DIRECTION('ref_axis',(0.996017466987621,-0.089158316805357,-1.17238054377005E-27));
#11158=DIRECTION('center_axis',(2.46563637061793E-17,5.67162995353388E-17,
1.));
#11159=DIRECTION('ref_axis',(-0.990654937187062,0.136392065117066,1.66902952191835E-17));
#11160=DIRECTION('center_axis',(-2.46563637061793E-17,-5.67162995353388E-17,
-1.));
#11161=DIRECTION('ref_axis',(-0.99065493718706,0.136392065117079,0.));
#11162=DIRECTION('center_axis',(-2.46563637061793E-17,-5.67162995353388E-17,
-1.));
#11163=DIRECTION('ref_axis',(-0.99065493718706,0.136392065117079,1.66902952191827E-17));
#11164=DIRECTION('center_axis',(-0.0891583168058793,-0.996017466987574,
5.86887448866932E-17));
#11165=DIRECTION('ref_axis',(0.996017466987574,-0.0891583168058793,2.42436373273487E-32));
#11166=DIRECTION('center_axis',(2.46563637061793E-17,5.67162995353388E-17,
1.));
#11167=DIRECTION('ref_axis',(-0.990654937187062,0.136392065117067,1.66902952191834E-17));
#11168=DIRECTION('center_axis',(-2.46563637061793E-17,-5.67162995353388E-17,
-1.));
#11169=DIRECTION('ref_axis',(-0.99065493718706,0.136392065117079,1.66902952191827E-17));
#11170=DIRECTION('center_axis',(-2.46563637061793E-17,-5.67162995353388E-17,
-1.));
#11171=DIRECTION('ref_axis',(0.99065493718706,-0.136392065117079,-1.66902952191827E-17));
#11172=DIRECTION('',(-2.46563637061793E-17,-5.67162995353388E-17,-1.));
#11173=DIRECTION('center_axis',(-2.46563637061793E-17,-5.67162995353388E-17,
-1.));
#11174=DIRECTION('ref_axis',(0.99065493718706,-0.136392065117079,-1.66902952191827E-17));
#11175=DIRECTION('',(-2.46563637061793E-17,-5.67162995353388E-17,-1.));
#11176=DIRECTION('center_axis',(-2.46563637061793E-17,-5.67162995353388E-17,
-1.));
#11177=DIRECTION('ref_axis',(-0.99065493718706,0.136392065117079,1.66902952191827E-17));
#11178=DIRECTION('',(-2.46563637061793E-17,-5.67162995353388E-17,-1.));
#11179=DIRECTION('',(-2.46563637061793E-17,-5.67162995353388E-17,-1.));
#11180=DIRECTION('center_axis',(-2.46563637061793E-17,-5.67162995353388E-17,
-1.));
#11181=DIRECTION('ref_axis',(-0.99065493718706,0.136392065117079,1.66902952191827E-17));
#11182=DIRECTION('center_axis',(-2.46563637061793E-17,-5.67162995353388E-17,
-1.));
#11183=DIRECTION('ref_axis',(0.99065493718706,-0.136392065117079,-1.66902952191827E-17));
#11184=DIRECTION('',(2.46563637061793E-17,5.67162995353388E-17,1.));
#11185=DIRECTION('center_axis',(-2.46563637061793E-17,-5.67162995353388E-17,
-1.));
#11186=DIRECTION('ref_axis',(0.99065493718706,-0.136392065117079,-1.66902952191827E-17));
#11187=DIRECTION('',(-2.46563637061793E-17,-5.67162995353388E-17,-1.));
#11188=DIRECTION('center_axis',(-2.46563637061793E-17,-5.67162995353388E-17,
-1.));
#11189=DIRECTION('ref_axis',(-0.99065493718706,0.136392065117079,1.66902952191827E-17));
#11190=DIRECTION('center_axis',(-2.46563637061793E-17,-5.67162995353388E-17,
-1.));
#11191=DIRECTION('ref_axis',(0.99065493718706,-0.136392065117079,-1.66902952191827E-17));
#11192=DIRECTION('center_axis',(0.272924859769355,-0.826517122498203,0.492322523491631));
#11193=DIRECTION('ref_axis',(-0.96059955766106,-0.262077780098513,0.0925404073905592));
#11194=DIRECTION('center_axis',(2.46563637061793E-17,5.67162995353388E-17,
1.));
#11195=DIRECTION('ref_axis',(-0.99065493718706,0.136392065117079,1.66902952191827E-17));
#11196=DIRECTION('',(-2.46563637061793E-17,-5.67162995353388E-17,-1.));
#11197=DIRECTION('center_axis',(-2.46563637061793E-17,-5.67162995353388E-17,
-1.));
#11198=DIRECTION('ref_axis',(-0.99065493718706,0.136392065117079,1.66902952191827E-17));
#11199=DIRECTION('center_axis',(0.272924859943062,-0.826517122450901,-0.492322523474746));
#11200=DIRECTION('ref_axis',(-0.960787153734946,-0.26023504479525,-0.0957380106243915));
#11201=DIRECTION('center_axis',(-2.46563637061793E-17,-5.67162995353388E-17,
-1.));
#11202=DIRECTION('ref_axis',(0.99065493718706,-0.136392065117079,-1.66902952191827E-17));
#11203=DIRECTION('',(2.46563637061793E-17,5.67162995353388E-17,1.));
#11204=DIRECTION('center_axis',(-2.46563637061793E-17,-5.67162995353388E-17,
-1.));
#11205=DIRECTION('ref_axis',(-0.99065493718706,0.136392065117079,1.66902952191827E-17));
#11206=DIRECTION('center_axis',(-2.46563637061793E-17,-5.67162995353388E-17,
-1.));
#11207=DIRECTION('ref_axis',(0.990654937187061,-0.136392065117078,-1.66902952191827E-17));
#11208=DIRECTION('',(2.46563637061793E-17,5.67162995353388E-17,1.));
#11209=DIRECTION('center_axis',(-2.46563637061793E-17,-5.67162995353388E-17,
-1.));
#11210=DIRECTION('ref_axis',(0.990654937187061,-0.136392065117078,-1.66902952191827E-17));
#11211=DIRECTION('',(-2.46563637061793E-17,-5.67162995353388E-17,-1.));
#11212=DIRECTION('center_axis',(-2.46563637061793E-17,-5.67162995353388E-17,
-1.));
#11213=DIRECTION('ref_axis',(-0.99065493718706,0.136392065117079,1.66902952191827E-17));
#11214=DIRECTION('',(2.46563637061793E-17,5.67162995353388E-17,1.));
#11215=DIRECTION('center_axis',(-2.46563637061793E-17,-5.67162995353388E-17,
-1.));
#11216=DIRECTION('ref_axis',(-0.99065493718706,0.136392065117079,1.66902952191827E-17));
#11217=DIRECTION('',(-2.46563637061793E-17,-5.67162995353388E-17,-1.));
#11218=DIRECTION('center_axis',(-2.46563637061793E-17,-5.67162995353388E-17,
-1.));
#11219=DIRECTION('ref_axis',(0.990654937187061,-0.136392065117077,-1.66902952191828E-17));
#11220=DIRECTION('center_axis',(-2.46563637061793E-17,-5.67162995353388E-17,
-1.));
#11221=DIRECTION('ref_axis',(-0.99065493718706,0.136392065117079,1.66902952191827E-17));
#11222=DIRECTION('center_axis',(-2.46563637061793E-17,-5.67162995353388E-17,
-1.));
#11223=DIRECTION('ref_axis',(-0.99065493718706,0.136392065117079,1.66902952191827E-17));
#11224=DIRECTION('center_axis',(-2.46563637061793E-17,-5.67162995353388E-17,
-1.));
#11225=DIRECTION('ref_axis',(-0.99065493718706,0.136392065117079,1.66902952191827E-17));
#11226=DIRECTION('center_axis',(-2.46563637061793E-17,-5.67162995353388E-17,
-1.));
#11227=DIRECTION('ref_axis',(-0.99065493718706,0.136392065117078,1.66902952191827E-17));
#11228=DIRECTION('center_axis',(-2.46563637061793E-17,-5.67162995353388E-17,
-1.));
#11229=DIRECTION('ref_axis',(-0.99065493718706,0.136392065117079,1.66902952191827E-17));
#11230=DIRECTION('center_axis',(2.46563637061793E-17,5.67162995353388E-17,
1.));
#11231=DIRECTION('ref_axis',(-0.990654937187061,0.136392065117072,1.66902952191831E-17));
#11232=DIRECTION('center_axis',(-2.46563637061793E-17,-5.67162995353388E-17,
-1.));
#11233=DIRECTION('ref_axis',(-0.99065493718706,0.136392065117079,1.66902952191827E-17));
#11234=DIRECTION('',(0.916721549040254,0.399526721916365,-4.52626971630091E-17));
#11235=DIRECTION('center_axis',(-2.46563637061793E-17,-5.67162995353388E-17,
-1.));
#11236=DIRECTION('ref_axis',(-0.99065493718706,0.136392065117079,1.66902952191826E-17));
#11237=DIRECTION('center_axis',(2.46563637061793E-17,5.67162995353388E-17,
1.));
#11238=DIRECTION('ref_axis',(-0.99065493718706,0.136392065117079,1.66902952191827E-17));
#11239=DIRECTION('center_axis',(2.46563637061793E-17,5.67162995353388E-17,
1.));
#11240=DIRECTION('ref_axis',(-0.99065493718706,0.136392065117079,1.66902952191827E-17));
#11241=DIRECTION('center_axis',(-2.46563637061793E-17,-5.67162995353388E-17,
-1.));
#11242=DIRECTION('ref_axis',(-0.99065493718706,0.136392065117079,1.66902952191827E-17));
#11243=DIRECTION('center_axis',(2.46563637061793E-17,5.67162995353388E-17,
1.));
#11244=DIRECTION('ref_axis',(-0.99065493718706,0.136392065117079,1.66902952191827E-17));
#11245=DIRECTION('center_axis',(-2.46563637061793E-17,-5.67162995353388E-17,
-1.));
#11246=DIRECTION('ref_axis',(-0.99065493718706,0.136392065117079,1.66902952191827E-17));
#11247=DIRECTION('center_axis',(-2.46563637061793E-17,-5.67162995353388E-17,
-1.));
#11248=DIRECTION('ref_axis',(-0.99065493718706,0.136392065117079,1.66902952191827E-17));
#11249=DIRECTION('center_axis',(2.46563637061793E-17,5.67162995353388E-17,
1.));
#11250=DIRECTION('ref_axis',(-0.990654937187061,0.136392065117077,1.66902952191828E-17));
#11251=DIRECTION('',(-0.916721549040254,-0.399526721916365,4.52626971630091E-17));
#11252=DIRECTION('center_axis',(2.46563637061793E-17,5.67162995353388E-17,
1.));
#11253=DIRECTION('ref_axis',(-0.990654937187061,0.136392065117077,1.66902952191828E-17));
#11254=DIRECTION('center_axis',(-2.46563637061793E-17,-5.67162995353388E-17,
-1.));
#11255=DIRECTION('ref_axis',(-0.99065493718706,0.136392065117079,1.66902952191827E-17));
#11256=DIRECTION('center_axis',(2.46563637061793E-17,5.67162995353388E-17,
1.));
#11257=DIRECTION('ref_axis',(-0.99065493718706,0.136392065117079,1.66902952191827E-17));
#11258=DIRECTION('center_axis',(2.46563637061793E-17,5.67162995353388E-17,
1.));
#11259=DIRECTION('ref_axis',(-0.99065493718706,0.136392065117078,1.66902952191827E-17));
#11260=DIRECTION('center_axis',(2.46563637061793E-17,5.67162995353388E-17,
1.));
#11261=DIRECTION('ref_axis',(-0.99065493718706,0.13639206511708,1.66902952191826E-17));
#11262=DIRECTION('center_axis',(-0.399526721916365,0.916721549040254,-4.21421777999594E-17));
#11263=DIRECTION('ref_axis',(-0.916721549040254,-0.399526721916365,4.52626971630091E-17));
#11264=DIRECTION('',(0.916721549040254,0.399526721916365,-4.52626971630091E-17));
#11265=DIRECTION('',(-0.916721549040254,-0.399526721916365,4.52626971630091E-17));
#11266=DIRECTION('',(-2.46563637061793E-17,-5.67162995353388E-17,-1.));
#11267=DIRECTION('',(-0.916721549040254,-0.399526721916365,4.52626971630091E-17));
#11268=DIRECTION('',(2.46563637061793E-17,5.67162995353388E-17,1.));
#11269=DIRECTION('',(-0.916721549040254,-0.399526721916365,4.52626971630091E-17));
#11270=DIRECTION('center_axis',(-2.46563637061793E-17,-5.67162995353388E-17,
-1.));
#11271=DIRECTION('ref_axis',(-0.99065493718706,0.136392065117079,1.66902952191827E-17));
#11272=DIRECTION('center_axis',(2.46563637061793E-17,5.67162995353388E-17,
1.));
#11273=DIRECTION('ref_axis',(-0.99065493718706,0.136392065117079,1.66902952191827E-17));
#11274=DIRECTION('',(2.46563637061793E-17,5.67162995353388E-17,1.));
#11275=DIRECTION('center_axis',(-2.46563637061793E-17,-5.67162995353388E-17,
-1.));
#11276=DIRECTION('ref_axis',(-0.99065493718706,0.136392065117079,1.66902952191827E-17));
#11277=DIRECTION('',(-2.46563637061793E-17,-5.67162995353388E-17,-1.));
#11278=DIRECTION('center_axis',(2.46563637061793E-17,5.67162995353388E-17,
1.));
#11279=DIRECTION('ref_axis',(0.99065493718706,-0.136392065117079,-1.66902952191827E-17));
#11280=DIRECTION('',(2.46563637061793E-17,5.67162995353388E-17,1.));
#11281=DIRECTION('center_axis',(2.46563637061793E-17,5.67162995353388E-17,
1.));
#11282=DIRECTION('ref_axis',(0.99065493718706,-0.136392065117079,-1.66902952191827E-17));
#11283=DIRECTION('center_axis',(-2.46563637061793E-17,-5.67162995353388E-17,
-1.));
#11284=DIRECTION('ref_axis',(0.960627000032841,-0.277841261888699,-7.92744046622962E-18));
#11285=DIRECTION('',(-2.46563637061793E-17,-5.67162995353388E-17,-1.));
#11286=DIRECTION('center_axis',(-2.46563637061793E-17,-5.67162995353388E-17,
-1.));
#11287=DIRECTION('ref_axis',(-0.99065493718706,0.136392065117079,1.66902952191827E-17));
#11288=DIRECTION('',(-2.46563637061793E-17,-5.67162995353388E-17,-1.));
#11289=DIRECTION('center_axis',(2.46563637061793E-17,5.67162995353388E-17,
1.));
#11290=DIRECTION('ref_axis',(-0.99065493718706,0.136392065117079,1.66902952191827E-17));
#11291=DIRECTION('center_axis',(-2.46563637061793E-17,-5.67162995353388E-17,
-1.));
#11292=DIRECTION('ref_axis',(-0.99065493718706,0.136392065117079,1.66902952191827E-17));
#11293=DIRECTION('center_axis',(2.46563637061793E-17,5.67162995353388E-17,
1.));
#11294=DIRECTION('ref_axis',(-0.99065493718706,0.136392065117079,1.66902952191827E-17));
#11295=DIRECTION('center_axis',(-2.46563637061793E-17,-5.67162995353388E-17,
-1.));
#11296=DIRECTION('ref_axis',(-0.99065493718706,0.136392065117079,1.66902952191827E-17));
#11297=DIRECTION('center_axis',(-0.136392065117079,-0.99065493718706,5.95492145178271E-17));
#11298=DIRECTION('ref_axis',(-2.46563637061793E-17,-5.67162995353388E-17,
-1.));
#11299=DIRECTION('',(-0.99065493718706,0.136392065117079,1.66902952191827E-17));
#11300=DIRECTION('',(-2.46563637061793E-17,-5.67162995353388E-17,-1.));
#11301=DIRECTION('',(-0.99065493718706,0.136392065117079,1.66902952191827E-17));
#11302=DIRECTION('center_axis',(-2.46563637061793E-17,-5.67162995353388E-17,
-1.));
#11303=DIRECTION('ref_axis',(-0.99065493718706,0.136392065117079,1.66902952191827E-17));
#11304=DIRECTION('center_axis',(0.494699854607087,-0.71082491082636,0.500000000000425));
#11305=DIRECTION('ref_axis',(0.285615094283029,-0.410394953572923,-0.866025403784193));
#11306=DIRECTION('center_axis',(2.46563637061793E-17,5.67162995353388E-17,
1.));
#11307=DIRECTION('ref_axis',(-0.990654937187061,0.136392065117072,1.66902952191831E-17));
#11308=DIRECTION('',(-2.46563637061793E-17,-5.67162995353388E-17,-1.));
#11309=DIRECTION('center_axis',(-2.46563637061793E-17,-5.67162995353388E-17,
-1.));
#11310=DIRECTION('ref_axis',(-0.99065493718706,0.136392065117079,1.66902952191827E-17));
#11311=DIRECTION('center_axis',(-0.494699854607571,0.710824910827106,0.499999999998885));
#11312=DIRECTION('ref_axis',(0.285615094167233,-0.410394953651635,0.866025403785083));
#11313=DIRECTION('center_axis',(-2.46563637061793E-17,-5.67162995353388E-17,
-1.));
#11314=DIRECTION('ref_axis',(-0.99065493718706,0.136392065117079,1.66902952191827E-17));
#11315=DIRECTION('center_axis',(2.46563637061793E-17,5.67162995353388E-17,
1.));
#11316=DIRECTION('ref_axis',(-0.990654937187061,0.136392065117077,1.66902952191828E-17));
#11317=DIRECTION('center_axis',(-2.46563637061793E-17,-5.67162995353388E-17,
-1.));
#11318=DIRECTION('ref_axis',(-0.99065493718706,0.136392065117079,1.66902952191827E-17));
#11319=DIRECTION('center_axis',(2.46563637061793E-17,5.67162995353388E-17,
1.));
#11320=DIRECTION('ref_axis',(0.99065493718706,-0.136392065117079,-1.66902952191827E-17));
#11321=DIRECTION('center_axis',(-2.46563637061793E-17,-5.67162995353388E-17,
-1.));
#11322=DIRECTION('ref_axis',(0.99065493718706,-0.136392065117079,-1.66902952191827E-17));
#11323=DIRECTION('center_axis',(2.46563637061793E-17,5.67162995353388E-17,
1.));
#11324=DIRECTION('ref_axis',(0.99065493718706,-0.136392065117079,-1.66902952191827E-17));
#11325=DIRECTION('center_axis',(2.46563637061793E-17,5.67162995353388E-17,
1.));
#11326=DIRECTION('ref_axis',(0.99065493718706,-0.136392065117079,-1.66902952191827E-17));
#11327=DIRECTION('',(-0.820789907224822,-0.57123018845109,5.26357569507164E-17));
#11328=DIRECTION('',(-0.78773404285246,-0.616015484976895,5.43607758286658E-17));
#11329=DIRECTION('',(0.616015484976899,-0.787734042852457,2.94886580823745E-17));
#11330=DIRECTION('',(-0.78773404285246,-0.616015484976895,5.43607758286658E-17));
#11331=DIRECTION('',(0.616015484976899,-0.787734042852457,2.94886580823745E-17));
#11332=DIRECTION('',(-0.78773404285246,-0.616015484976895,5.43607758286658E-17));
#11333=DIRECTION('',(0.616015484976899,-0.787734042852457,2.94886580823745E-17));
#11334=DIRECTION('',(-0.78773404285246,-0.616015484976895,5.43607758286658E-17));
#11335=DIRECTION('',(0.616015484976899,-0.787734042852457,2.94886580823745E-17));
#11336=DIRECTION('',(-0.78773404285246,-0.616015484976895,5.43607758286658E-17));
#11337=DIRECTION('',(0.616015484976899,-0.787734042852457,2.94886580823745E-17));
#11338=DIRECTION('',(-0.78773404285246,-0.616015484976895,5.43607758286658E-17));
#11339=DIRECTION('',(0.616015484976899,-0.787734042852457,2.94886580823745E-17));
#11340=DIRECTION('',(-0.78773404285246,-0.616015484976895,5.43607758286658E-17));
#11341=DIRECTION('',(0.616015484976899,-0.787734042852457,2.94886580823745E-17));
#11342=DIRECTION('',(-0.78773404285246,-0.616015484976895,5.43607758286658E-17));
#11343=DIRECTION('',(0.616015484976899,-0.787734042852457,2.94886580823745E-17));
#11344=DIRECTION('',(-0.78773404285246,-0.616015484976895,5.43607758286658E-17));
#11345=DIRECTION('',(0.616015484976899,-0.787734042852457,2.94886580823745E-17));
#11346=DIRECTION('center_axis',(2.46563637061793E-17,5.67162995353388E-17,
1.));
#11347=DIRECTION('ref_axis',(0.99065493718706,-0.136392065117079,-1.66902952191827E-17));
#11348=DIRECTION('',(0.499271281878494,0.026984941938175,-0.866025403784438));
#11349=DIRECTION('center_axis',(-2.46563637061793E-17,-5.67162995353388E-17,
-1.));
#11350=DIRECTION('ref_axis',(-0.99065493718706,0.136392065117079,1.66902952191827E-17));
#11351=DIRECTION('',(0.498008733493835,-0.0445791584024184,-0.866025403784438));
#11352=DIRECTION('center_axis',(2.46563637061793E-17,5.67162995353388E-17,
1.));
#11353=DIRECTION('ref_axis',(-0.96497141127135,0.262355056038528,8.91287813947976E-18));
#11354=DIRECTION('center_axis',(-0.494699854607216,0.710824910826568,-0.500000000000001));
#11355=DIRECTION('ref_axis',(-0.820789907224822,-0.57123018845109,2.73331257345188E-17));
#11356=DIRECTION('center_axis',(2.46563637061793E-17,5.67162995353388E-17,
1.));
#11357=DIRECTION('ref_axis',(0.99065493718706,-0.136392065117079,-1.66902952191827E-17));
#11358=DIRECTION('center_axis',(-0.457286527460412,0.756141387770446,0.468123096528875));
#11359=DIRECTION('ref_axis',(-0.887435897002915,-0.422223938468998,-0.184890439164279));
#11360=DIRECTION('center_axis',(-2.46563637061793E-17,-5.67162995353388E-17,
-1.));
#11361=DIRECTION('ref_axis',(0.990654937187061,-0.136392065117078,-1.66902952191827E-17));
#11362=DIRECTION('center_axis',(-2.46563637061793E-17,-5.67162995353388E-17,
-1.));
#11363=DIRECTION('ref_axis',(0.99065493718706,-0.136392065117079,-1.66902952191827E-17));
#11364=DIRECTION('center_axis',(2.46563637061793E-17,5.67162995353388E-17,
1.));
#11365=DIRECTION('ref_axis',(0.990654937187061,-0.136392065117078,-1.66902952191827E-17));
#11366=DIRECTION('center_axis',(-0.457286527428201,0.756141387785753,-0.468123096535616));
#11367=DIRECTION('ref_axis',(-0.887545517051143,-0.421261555860625,0.186552021474719));
#11368=DIRECTION('center_axis',(-2.46563637061793E-17,-5.67162995353388E-17,
-1.));
#11369=DIRECTION('ref_axis',(0.990654937187061,-0.136392065117077,-1.66902952191827E-17));
#11370=DIRECTION('',(-0.499271281878494,-0.0269849419381751,-0.866025403784438));
#11371=DIRECTION('center_axis',(-0.494699854607216,0.710824910826568,0.500000000000001));
#11372=DIRECTION('ref_axis',(-0.820789907224822,-0.57123018845109,4.76302227498196E-17));
#11373=DIRECTION('',(-0.820789907224822,-0.57123018845109,5.26357569507164E-17));
#11374=DIRECTION('center_axis',(-2.46563637061793E-17,-5.67162995353388E-17,
-1.));
#11375=DIRECTION('ref_axis',(-0.964971411271351,0.262355056038526,8.91287813947992E-18));
#11376=DIRECTION('center_axis',(2.46563637061793E-17,5.67162995353388E-17,
1.));
#11377=DIRECTION('ref_axis',(0.99065493718706,-0.136392065117079,-1.66902952191827E-17));
#11378=DIRECTION('',(-0.498008733493835,0.0445791584024182,-0.866025403784438));
#11379=DIRECTION('center_axis',(-2.46563637061793E-17,-5.67162995353388E-17,
-1.));
#11380=DIRECTION('ref_axis',(0.99065493718706,-0.136392065117079,-1.66902952191827E-17));
#11381=DIRECTION('center_axis',(2.46563637061793E-17,5.67162995353388E-17,
1.));
#11382=DIRECTION('ref_axis',(-0.99065493718706,0.136392065117079,1.66902952191827E-17));
#11383=DIRECTION('center_axis',(2.46563637061793E-17,5.67162995353388E-17,
1.));
#11384=DIRECTION('ref_axis',(0.99065493718706,-0.136392065117079,-1.66902952191827E-17));
#11385=DIRECTION('center_axis',(2.46563637061793E-17,5.67162995353388E-17,
1.));
#11386=DIRECTION('ref_axis',(0.99065493718706,-0.136392065117079,-1.66902952191827E-17));
#11387=DIRECTION('',(0.616015484976889,-0.787734042852464,2.94886580823751E-17));
#11388=DIRECTION('',(-0.787734042852462,-0.616015484976892,5.43607758286657E-17));
#11389=DIRECTION('',(0.616015484976889,-0.787734042852464,2.94886580823751E-17));
#11390=DIRECTION('',(-0.787734042852462,-0.616015484976892,5.43607758286657E-17));
#11391=DIRECTION('',(0.616015484976889,-0.787734042852464,2.94886580823751E-17));
#11392=DIRECTION('',(-0.787734042852462,-0.616015484976892,5.43607758286657E-17));
#11393=DIRECTION('',(0.616015484976889,-0.787734042852464,2.94886580823751E-17));
#11394=DIRECTION('',(-0.787734042852462,-0.616015484976892,5.43607758286657E-17));
#11395=DIRECTION('',(0.616015484976889,-0.787734042852464,2.94886580823751E-17));
#11396=DIRECTION('',(-0.787734042852462,-0.616015484976892,5.43607758286657E-17));
#11397=DIRECTION('',(0.616015484976889,-0.787734042852464,2.94886580823751E-17));
#11398=DIRECTION('',(-0.787734042852462,-0.616015484976892,5.43607758286657E-17));
#11399=DIRECTION('',(0.616015484976889,-0.787734042852464,2.94886580823751E-17));
#11400=DIRECTION('',(-0.787734042852462,-0.616015484976892,5.43607758286657E-17));
#11401=DIRECTION('',(0.616015484976889,-0.787734042852464,2.94886580823751E-17));
#11402=DIRECTION('',(-0.787734042852462,-0.616015484976892,5.43607758286657E-17));
#11403=DIRECTION('',(0.616015484976889,-0.787734042852464,2.94886580823751E-17));
#11404=DIRECTION('',(-0.787734042852462,-0.616015484976892,5.43607758286657E-17));
#11405=DIRECTION('center_axis',(-2.46563637061793E-17,-5.67162995353388E-17,
-1.));
#11406=DIRECTION('ref_axis',(-0.99065493718706,0.136392065117079,0.));
#11407=DIRECTION('center_axis',(0.0539698838763491,-0.998542563756985,5.53029380587908E-17));
#11408=DIRECTION('ref_axis',(0.998542563756985,0.0539698838763491,-5.40660864842981E-32));
#11409=DIRECTION('center_axis',(-2.46563637061793E-17,-5.67162995353388E-17,
-1.));
#11410=DIRECTION('ref_axis',(-0.99065493718706,0.136392065117079,0.));
#11411=DIRECTION('center_axis',(-2.46563637061793E-17,-5.67162995353388E-17,
-1.));
#11412=DIRECTION('ref_axis',(-0.99065493718706,0.136392065117079,0.));
#11413=DIRECTION('center_axis',(0.0539698838763491,-0.998542563756986,5.53029380587908E-17));
#11414=DIRECTION('ref_axis',(0.998542563756985,0.0539698838763491,-5.4506213724986E-32));
#11415=DIRECTION('center_axis',(-2.46563637061793E-17,-5.67162995353388E-17,
-1.));
#11416=DIRECTION('ref_axis',(-0.99065493718706,0.136392065117079,0.));
#11417=DIRECTION('center_axis',(-2.46563637061793E-17,-5.67162995353388E-17,
-1.));
#11418=DIRECTION('ref_axis',(-0.99065493718706,0.136392065117079,1.66902952191827E-17));
#11419=DIRECTION('center_axis',(2.46563637061793E-17,5.67162995353388E-17,
1.));
#11420=DIRECTION('ref_axis',(-0.99065493718706,0.13639206511708,1.66902952191826E-17));
#11421=DIRECTION('center_axis',(-2.46563637061793E-17,-5.67162995353388E-17,
-1.));
#11422=DIRECTION('ref_axis',(0.990654937187061,-0.136392065117077,-1.66902952191828E-17));
#11423=DIRECTION('center_axis',(-0.99065493718706,0.136392065117079,1.66902952191827E-17));
#11424=DIRECTION('ref_axis',(-0.136392065117079,-0.99065493718706,5.95492145178272E-17));
#11425=DIRECTION('',(0.136392065117079,0.99065493718706,-5.95492145178271E-17));
#11426=DIRECTION('',(0.136392065117079,0.99065493718706,-5.95492145178271E-17));
#11427=DIRECTION('',(-2.46563637061793E-17,-5.67162995353388E-17,-1.));
#11428=DIRECTION('center_axis',(2.46563637061793E-17,5.67162995353388E-17,
1.));
#11429=DIRECTION('ref_axis',(0.99065493718706,-0.136392065117079,-1.66902952191827E-17));
#11430=DIRECTION('',(0.663255030075764,-0.748393456063852,2.60926501729039E-17));
#11431=DIRECTION('center_axis',(2.46563637061793E-17,5.67162995353388E-17,
1.));
#11432=DIRECTION('ref_axis',(0.99065493718706,-0.136392065117079,-1.66902952191827E-17));
#11433=DIRECTION('center_axis',(2.46563637061793E-17,5.67162995353388E-17,
1.));
#11434=DIRECTION('ref_axis',(0.99065493718706,-0.136392065117079,-1.66902952191827E-17));
#11435=DIRECTION('center_axis',(2.46563637061793E-17,5.67162995353388E-17,
1.));
#11436=DIRECTION('ref_axis',(0.99065493718706,-0.136392065117079,-1.66902952191827E-17));
#11437=DIRECTION('',(0.663255030075764,-0.748393456063852,2.60926501729039E-17));
#11438=DIRECTION('center_axis',(-2.46563637061793E-17,-5.67162995353388E-17,
-1.));
#11439=DIRECTION('ref_axis',(-0.99065493718706,0.136392065117079,1.66902952191827E-17));
#11440=DIRECTION('',(-2.46563637061793E-17,-5.67162995353388E-17,-1.));
#11441=DIRECTION('center_axis',(0.748393456063852,0.663255030075765,-5.6070032202132E-17));
#11442=DIRECTION('ref_axis',(-0.663255030075765,0.748393456063852,-2.60926501729039E-17));
#11443=DIRECTION('center_axis',(-0.787734042852464,-0.61601548497689,5.43607758286656E-17));
#11444=DIRECTION('ref_axis',(0.61601548497689,-0.787734042852464,2.94886580823751E-17));
#11445=DIRECTION('',(-2.46563637061793E-17,-5.67162995353388E-17,-1.));
#11446=DIRECTION('',(2.46563637061793E-17,5.67162995353388E-17,1.));
#11447=DIRECTION('center_axis',(-0.616015484976892,0.787734042852462,-2.9488658082375E-17));
#11448=DIRECTION('ref_axis',(-0.787734042852462,-0.616015484976892,5.43607758286657E-17));
#11449=DIRECTION('center_axis',(-0.616015484976892,0.787734042852462,-2.9488658082375E-17));
#11450=DIRECTION('ref_axis',(-0.787734042852462,-0.616015484976892,5.43607758286657E-17));
#11451=DIRECTION('',(2.46563637061793E-17,5.67162995353388E-17,1.));
#11452=DIRECTION('center_axis',(-0.616015484976892,0.787734042852462,-2.9488658082375E-17));
#11453=DIRECTION('ref_axis',(-0.787734042852462,-0.616015484976892,5.43607758286657E-17));
#11454=DIRECTION('',(2.46563637061793E-17,5.67162995353388E-17,1.));
#11455=DIRECTION('',(-2.46563637061793E-17,-5.67162995353388E-17,-1.));
#11456=DIRECTION('center_axis',(-0.616015484976892,0.787734042852462,-2.9488658082375E-17));
#11457=DIRECTION('ref_axis',(-0.787734042852462,-0.616015484976892,5.43607758286657E-17));
#11458=DIRECTION('',(2.46563637061793E-17,5.67162995353388E-17,1.));
#11459=DIRECTION('',(-2.46563637061793E-17,-5.67162995353388E-17,-1.));
#11460=DIRECTION('center_axis',(-0.616015484976892,0.787734042852462,-2.9488658082375E-17));
#11461=DIRECTION('ref_axis',(-0.787734042852462,-0.616015484976892,5.43607758286657E-17));
#11462=DIRECTION('',(2.46563637061793E-17,5.67162995353388E-17,1.));
#11463=DIRECTION('',(-2.46563637061793E-17,-5.67162995353388E-17,-1.));
#11464=DIRECTION('center_axis',(-0.616015484976892,0.787734042852462,-2.9488658082375E-17));
#11465=DIRECTION('ref_axis',(-0.787734042852462,-0.616015484976892,5.43607758286657E-17));
#11466=DIRECTION('',(2.46563637061793E-17,5.67162995353388E-17,1.));
#11467=DIRECTION('',(-2.46563637061793E-17,-5.67162995353388E-17,-1.));
#11468=DIRECTION('center_axis',(-0.616015484976892,0.787734042852462,-2.9488658082375E-17));
#11469=DIRECTION('ref_axis',(-0.787734042852462,-0.616015484976892,5.43607758286657E-17));
#11470=DIRECTION('',(2.46563637061793E-17,5.67162995353388E-17,1.));
#11471=DIRECTION('',(-2.46563637061793E-17,-5.67162995353388E-17,-1.));
#11472=DIRECTION('center_axis',(-0.787734042852464,-0.61601548497689,5.43607758286656E-17));
#11473=DIRECTION('ref_axis',(0.61601548497689,-0.787734042852464,2.94886580823751E-17));
#11474=DIRECTION('center_axis',(-0.787734042852464,-0.61601548497689,5.43607758286656E-17));
#11475=DIRECTION('ref_axis',(0.61601548497689,-0.787734042852464,2.94886580823751E-17));
#11476=DIRECTION('center_axis',(-0.787734042852464,-0.61601548497689,5.43607758286656E-17));
#11477=DIRECTION('ref_axis',(0.61601548497689,-0.787734042852464,2.94886580823751E-17));
#11478=DIRECTION('center_axis',(-0.787734042852464,-0.61601548497689,5.43607758286656E-17));
#11479=DIRECTION('ref_axis',(0.61601548497689,-0.787734042852464,2.94886580823751E-17));
#11480=DIRECTION('center_axis',(-0.787734042852464,-0.61601548497689,5.43607758286656E-17));
#11481=DIRECTION('ref_axis',(0.61601548497689,-0.787734042852464,2.94886580823751E-17));
#11482=DIRECTION('center_axis',(-0.787734042852464,-0.61601548497689,5.43607758286656E-17));
#11483=DIRECTION('ref_axis',(0.61601548497689,-0.787734042852464,2.94886580823751E-17));
#11484=DIRECTION('center_axis',(-0.616015484976892,0.787734042852462,-2.9488658082375E-17));
#11485=DIRECTION('ref_axis',(-0.787734042852462,-0.616015484976892,5.43607758286657E-17));
#11486=DIRECTION('',(2.46563637061793E-17,5.67162995353388E-17,1.));
#11487=DIRECTION('center_axis',(-0.787734042852464,-0.61601548497689,5.43607758286656E-17));
#11488=DIRECTION('ref_axis',(0.61601548497689,-0.787734042852464,2.94886580823751E-17));
#11489=DIRECTION('center_axis',(-0.787734042852464,-0.61601548497689,5.43607758286656E-17));
#11490=DIRECTION('ref_axis',(0.61601548497689,-0.787734042852464,2.94886580823751E-17));
#11491=DIRECTION('',(2.46563637061793E-17,5.67162995353388E-17,1.));
#11492=DIRECTION('center_axis',(-0.616015484976892,0.787734042852462,-2.9488658082375E-17));
#11493=DIRECTION('ref_axis',(-0.787734042852462,-0.616015484976892,5.43607758286657E-17));
#11494=DIRECTION('center_axis',(-2.46563637061793E-17,-5.67162995353388E-17,
-1.));
#11495=DIRECTION('ref_axis',(-0.99065493718706,0.136392065117079,0.));
#11496=DIRECTION('center_axis',(-0.989544138268184,0.144230365800956,1.62183475475996E-17));
#11497=DIRECTION('ref_axis',(-0.144230365800956,-0.989544138268184,2.55261967089169E-32));
#11498=DIRECTION('center_axis',(-0.368026070136058,0.929815471854609,-4.36615081756679E-17));
#11499=DIRECTION('ref_axis',(-0.929815471854609,-0.368026070136058,5.79450330564664E-32));
#11500=DIRECTION('center_axis',(-2.46563637061793E-17,-5.67162995353388E-17,
-1.));
#11501=DIRECTION('ref_axis',(-0.99065493718706,0.136392065117079,0.));
#11502=DIRECTION('center_axis',(-0.916721549040254,-0.399526721916366,4.52626971630092E-17));
#11503=DIRECTION('ref_axis',(0.399526721916366,-0.916721549040254,2.21817733744602E-31));
#11504=DIRECTION('center_axis',(-0.916721549040254,-0.399526721916365,4.52626971630091E-17));
#11505=DIRECTION('ref_axis',(0.399526721916365,-0.916721549040254,2.67901058084089E-31));
#11506=DIRECTION('center_axis',(-2.46563637061793E-17,-5.67162995353388E-17,
-1.));
#11507=DIRECTION('ref_axis',(-0.99065493718706,0.136392065117079,0.));
#11508=DIRECTION('center_axis',(0.157680228170735,0.98749022559417,-5.98946124780692E-17));
#11509=DIRECTION('ref_axis',(-0.98749022559417,0.157680228170735,2.28905066400457E-31));
#11510=DIRECTION('center_axis',(-2.46563637061793E-17,-5.67162995353388E-17,
-1.));
#11511=DIRECTION('ref_axis',(-0.99065493718706,0.136392065117079,0.));
#11512=DIRECTION('center_axis',(0.708008807113558,0.706203603112896,-5.75101777424565E-17));
#11513=DIRECTION('ref_axis',(-0.706203603112896,0.708008807113558,-2.20184166772643E-31));
#11514=DIRECTION('center_axis',(0.585101922340639,0.486005175527197,-0.649195432696555));
#11515=DIRECTION('ref_axis',(0.103177631811544,0.749408921066127,0.654018841716556));
#11516=DIRECTION('center_axis',(-2.46563637061793E-17,-5.67162995353388E-17,
-1.));
#11517=DIRECTION('ref_axis',(-0.99065493718706,0.136392065117079,0.));
#11518=DIRECTION('center_axis',(-0.989544138268184,0.144230365800956,1.62183475475996E-17));
#11519=DIRECTION('ref_axis',(-0.144230365800956,-0.989544138268184,2.55261967089169E-32));
#11520=DIRECTION('center_axis',(-0.368026070136058,0.929815471854609,-4.36615081756679E-17));
#11521=DIRECTION('ref_axis',(-0.929815471854609,-0.368026070136058,5.79450330564664E-32));
#11522=DIRECTION('center_axis',(-2.46563637061793E-17,-5.67162995353388E-17,
-1.));
#11523=DIRECTION('ref_axis',(-0.99065493718706,0.136392065117079,0.));
#11524=DIRECTION('center_axis',(-0.916721549040254,-0.399526721916366,4.52626971630092E-17));
#11525=DIRECTION('ref_axis',(0.399526721916366,-0.916721549040254,2.21817733744602E-31));
#11526=DIRECTION('center_axis',(0.916721549040254,0.399526721916365,-4.52626971630091E-17));
#11527=DIRECTION('ref_axis',(-0.399526721916365,0.916721549040254,-2.67901058084089E-31));
#11528=DIRECTION('center_axis',(-2.46563637061793E-17,-5.67162995353388E-17,
-1.));
#11529=DIRECTION('ref_axis',(-0.99065493718706,0.136392065117079,0.));
#11530=DIRECTION('center_axis',(0.157680228170735,0.98749022559417,-5.98946124780692E-17));
#11531=DIRECTION('ref_axis',(-0.98749022559417,0.157680228170735,2.28905066400457E-31));
#11532=DIRECTION('center_axis',(-2.46563637061793E-17,-5.67162995353388E-17,
-1.));
#11533=DIRECTION('ref_axis',(-0.99065493718706,0.136392065117079,0.));
#11534=DIRECTION('center_axis',(0.708008807113593,0.70620360311286,-1.88773974627704E-13));
#11535=DIRECTION('ref_axis',(-0.70620360311286,0.708008807113593,9.97021596630967E-28));
#11536=DIRECTION('center_axis',(0.585101922340452,0.486005175526929,0.649195432696924));
#11537=DIRECTION('ref_axis',(-0.103177631811576,-0.749408921066484,0.654018841716142));
#11538=DIRECTION('center_axis',(0.0527382027779713,-0.500066547561434,0.864379621449822));
#11539=DIRECTION('ref_axis',(-0.118759166955581,-0.862582108275705,-0.491780811690185));
#11540=DIRECTION('center_axis',(0.117812303642623,-0.993035881079037,5.34164974729424E-17));
#11541=DIRECTION('ref_axis',(0.993035881079037,0.117812303642623,-1.38256563133947E-31));
#11542=DIRECTION('center_axis',(-2.46563637061793E-17,-5.67162995353388E-17,
-1.));
#11543=DIRECTION('ref_axis',(-0.99065493718706,0.136392065117079,0.));
#11544=DIRECTION('center_axis',(0.231338519431928,-0.972873316227269,4.94738077387215E-17));
#11545=DIRECTION('ref_axis',(0.972873316227269,0.231338519431928,-7.26928861059308E-32));
#11546=DIRECTION('center_axis',(-2.46563637061793E-17,-5.67162995353388E-17,
-1.));
#11547=DIRECTION('ref_axis',(-0.99065493718706,0.136392065117079,0.));
#11548=DIRECTION('center_axis',(0.910390173593427,-0.413750808850605,1.01950357310838E-18));
#11549=DIRECTION('ref_axis',(0.413750808850605,0.910390173593427,3.00458402755694E-33));
#11550=DIRECTION('center_axis',(-2.46563637061793E-17,-5.67162995353388E-17,
-1.));
#11551=DIRECTION('ref_axis',(0.960627000032841,-0.2778412618887,0.));
#11552=DIRECTION('center_axis',(-0.990695324577823,0.136098397711516,1.67079467539161E-17));
#11553=DIRECTION('ref_axis',(-0.136098397711516,-0.990695324577823,-3.08356560958003E-32));
#11554=DIRECTION('center_axis',(0.,0.,1.));
#11555=DIRECTION('ref_axis',(-0.990695324577823,0.136098397711516,0.));
#11556=DIRECTION('center_axis',(2.46563637061793E-17,5.67162995353388E-17,
1.));
#11557=DIRECTION('ref_axis',(0.99065493718706,-0.136392065117079,-1.66902952191826E-17));
#11558=DIRECTION('center_axis',(-2.46563637061793E-17,-5.67162995353388E-17,
-1.));
#11559=DIRECTION('ref_axis',(-0.99065493718706,0.13639206511708,1.66902952191826E-17));
#11560=DIRECTION('center_axis',(2.46563637061793E-17,5.67162995353388E-17,
1.));
#11561=DIRECTION('ref_axis',(0.99065493718706,-0.136392065117079,-1.66902952191826E-17));
#11562=DIRECTION('center_axis',(0.,0.,1.));
#11563=DIRECTION('ref_axis',(-0.990695324577823,0.136098397711516,0.));
#11564=DIRECTION('center_axis',(0.990695324577823,-0.136098397711516,-1.67079467539161E-17));
#11565=DIRECTION('ref_axis',(0.136098397711516,0.990695324577823,3.19570144840529E-32));
#11566=DIRECTION('center_axis',(-2.46563637061793E-17,-5.67162995353388E-17,
-1.));
#11567=DIRECTION('ref_axis',(0.960627000032841,-0.2778412618887,0.));
#11568=DIRECTION('center_axis',(-0.910390173593428,0.413750808850603,-1.01950357310826E-18));
#11569=DIRECTION('ref_axis',(-0.413750808850603,-0.910390173593428,-1.1114346208305E-33));
#11570=DIRECTION('center_axis',(-2.46563637061793E-17,-5.67162995353388E-17,
-1.));
#11571=DIRECTION('ref_axis',(-0.99065493718706,0.136392065117079,0.));
#11572=DIRECTION('center_axis',(-0.231338519431928,0.972873316227269,-4.94738077387215E-17));
#11573=DIRECTION('ref_axis',(-0.972873316227269,-0.231338519431928,7.26928861059308E-32));
#11574=DIRECTION('center_axis',(-2.46563637061793E-17,-5.67162995353388E-17,
-1.));
#11575=DIRECTION('ref_axis',(-0.99065493718706,0.136392065117079,0.));
#11576=DIRECTION('center_axis',(-0.117812303642623,0.993035881079037,-5.34164974729424E-17));
#11577=DIRECTION('ref_axis',(-0.993035881079037,-0.117812303642623,1.38256563133947E-31));
#11578=DIRECTION('center_axis',(-0.0527382027779737,0.500066547561435,0.864379621449822));
#11579=DIRECTION('ref_axis',(-0.118759166955581,-0.862582108275704,0.491780811690186));
#44354=CARTESIAN_POINT('',(0.,0.,0.));
#44355=CARTESIAN_POINT('Origin',(-69.9391102914966,14.1820463536532,177.985485069079));
#44356=CARTESIAN_POINT('',(-73.3730842378033,18.9797356866641,178.485485069079));
#44357=CARTESIAN_POINT('',(-67.58190263219,8.77338921431569,178.485485069079));
#44358=CARTESIAN_POINT('Origin',(-69.9391102914966,14.1820463536532,178.485485069079));
#44359=CARTESIAN_POINT('',(-73.6640989790157,19.3863195284447,177.985485069079));
#44360=CARTESIAN_POINT('Origin',(-73.3730842378033,18.9797356866641,177.985485069079));
#44361=CARTESIAN_POINT('',(-67.3821392712318,8.31502843979556,177.985485069079));
#44362=CARTESIAN_POINT('Origin',(-69.9391102914966,14.1820463536532,177.985485069079));
#44363=CARTESIAN_POINT('Origin',(-67.58190263219,8.77338921431569,177.985485069079));
#44364=CARTESIAN_POINT('Origin',(-69.9391102914966,14.1820463536532,173.985485069079));
#44365=CARTESIAN_POINT('',(-73.6640989790157,19.3863195284447,173.985485069079));
#44366=CARTESIAN_POINT('',(-67.3821392712318,8.31502843979556,173.985485069079));
#44367=CARTESIAN_POINT('Origin',(-69.9391102914966,14.1820463536532,173.985485069079));
#44368=CARTESIAN_POINT('',(-73.3730842378033,18.9797356866641,173.485485069079));
#44369=CARTESIAN_POINT('Origin',(-73.3730842378033,18.9797356866641,173.985485069079));
#44370=CARTESIAN_POINT('',(-67.58190263219,8.77338921431569,173.485485069079));
#44371=CARTESIAN_POINT('Origin',(-69.9391102914966,14.1820463536532,173.485485069079));
#44372=CARTESIAN_POINT('Origin',(-67.58190263219,8.77338921431569,173.985485069079));
#44373=CARTESIAN_POINT('Origin',(-55.2165279528263,6.30034797823479,177.185485069079));
#44374=CARTESIAN_POINT('',(-53.7305455470457,6.09575988055917,177.185485069079));
#44375=CARTESIAN_POINT('Origin',(-55.2165279528263,6.30034797823479,177.185485069079));
#44376=CARTESIAN_POINT('',(-53.7305455470457,6.09575988055917,174.785485069079));
#44377=CARTESIAN_POINT('',(-53.7305455470457,6.09575988055917,177.185485069079));
#44378=CARTESIAN_POINT('Origin',(-55.2165279528263,6.30034797823479,174.785485069079));
#44379=CARTESIAN_POINT('Origin',(-69.9391102914966,14.1820463536532,171.985485069079));
#44380=CARTESIAN_POINT('',(-71.9204201658707,14.4548304838874,173.485485069079));
#44381=CARTESIAN_POINT('Origin',(-69.9391102914966,14.1820463536532,173.485485069079));
#44382=CARTESIAN_POINT('',(-71.9204201658707,14.4548304838874,178.485485069079));
#44383=CARTESIAN_POINT('',(-71.9204201658707,14.4548304838874,171.985485069079));
#44384=CARTESIAN_POINT('Origin',(-69.9391102914966,14.1820463536532,178.485485069079));
#44385=CARTESIAN_POINT('Origin',(-38.9776940652673,8.40516957928931,171.985485069079));
#44386=CARTESIAN_POINT('',(-40.9590039396414,8.67795370952346,173.485485069079));
#44387=CARTESIAN_POINT('Origin',(-38.9776940652673,8.40516957928931,173.485485069079));
#44388=CARTESIAN_POINT('',(-40.9590039396414,8.67795370952346,178.485485069079));
#44389=CARTESIAN_POINT('',(-40.9590039396414,8.67795370952346,171.985485069079));
#44390=CARTESIAN_POINT('Origin',(-38.9776940652673,8.40516957928931,178.485485069079));
#44391=CARTESIAN_POINT('Origin',(-36.5934363437889,54.2142642791517,172.485485069079));
#44392=CARTESIAN_POINT('',(-50.6604618554941,55.4734714302896,172.985485069079));
#44393=CARTESIAN_POINT('',(-49.7994785223376,59.2209856988867,172.985485069079));
#44394=CARTESIAN_POINT('Origin',(-36.5934363437889,54.2142642791517,172.985485069079));
#44395=CARTESIAN_POINT('',(-51.5230382845183,55.5506847976022,173.485485069079));
#44396=CARTESIAN_POINT('Origin',(-51.5230382845184,55.5506847976013,172.485485069079));
#44397=CARTESIAN_POINT('',(-51.2438457370578,57.3835762739523,173.485485069079));
#44398=CARTESIAN_POINT('Origin',(-36.5934363437889,54.2142642791517,173.485485069079));
#44399=CARTESIAN_POINT('Ctrl Pts',(-51.2438457370578,57.3835762739523,173.485485069079));
#44400=CARTESIAN_POINT('Ctrl Pts',(-51.1924620128878,57.4555875576865,173.485485069079));
#44401=CARTESIAN_POINT('Ctrl Pts',(-51.1407466430462,57.5273107046625,173.48365231973));
#44402=CARTESIAN_POINT('Ctrl Pts',(-51.088733797749,57.5986654010425,173.480047403934));
#44403=CARTESIAN_POINT('Ctrl Pts',(-51.0368178468029,57.6698871712776,173.476449203709));
#44404=CARTESIAN_POINT('Ctrl Pts',(-50.9846044885947,57.7407416201286,173.471085313099));
#44405=CARTESIAN_POINT('Ctrl Pts',(-50.9321306284918,57.8111529948007,173.463964962461));
#44406=CARTESIAN_POINT('Ctrl Pts',(-50.8803221459752,57.8806715411113,173.456934899095));
#44407=CARTESIAN_POINT('Ctrl Pts',(-50.8282588216532,57.9497578739147,173.448192322867));
#44408=CARTESIAN_POINT('Ctrl Pts',(-50.7759933930428,58.0183471515507,173.437699729118));
#44409=CARTESIAN_POINT('Ctrl Pts',(-50.7252918589377,58.0848840898626,173.427521096436));
#44410=CARTESIAN_POINT('Ctrl Pts',(-50.6743994664868,58.1509529687663,173.41569511002));
#44411=CARTESIAN_POINT('Ctrl Pts',(-50.6233919622077,58.2165066509814,173.402149742799));
#44412=CARTESIAN_POINT('Ctrl Pts',(-50.5902712724658,58.2590726067317,173.393354332956));
#44413=CARTESIAN_POINT('Ctrl Pts',(-50.5571026313059,58.3014215878905,173.383833224202));
#44414=CARTESIAN_POINT('Ctrl Pts',(-50.5239152725159,58.3435445498383,173.373559351834));
#44415=CARTESIAN_POINT('Ctrl Pts',(-50.4846204001192,58.3934194562805,173.361394765124));
#44416=CARTESIAN_POINT('Ctrl Pts',(-50.4452379534982,58.4430651051017,173.348160519015));
#44417=CARTESIAN_POINT('Ctrl Pts',(-50.4057859651512,58.4923925183112,173.333744171839));
#44418=CARTESIAN_POINT('Ctrl Pts',(-50.3671961550944,58.5406419370631,173.319642877519));
#44419=CARTESIAN_POINT('Ctrl Pts',(-50.3285393960941,58.5885865961815,173.304410206274));
#44420=CARTESIAN_POINT('Ctrl Pts',(-50.2898712506386,58.6361573428422,173.287913558918));
#44421=CARTESIAN_POINT('Ctrl Pts',(-50.2524971554251,58.6821361089333,173.271968980721));
#44422=CARTESIAN_POINT('Ctrl Pts',(-50.2151121387377,58.7277653266149,173.254843160663));
#44423=CARTESIAN_POINT('Ctrl Pts',(-50.1778078229766,58.7729996473115,173.23639656982));
#44424=CARTESIAN_POINT('Ctrl Pts',(-50.1707542187054,58.7815526790764,173.232908636875));
#44425=CARTESIAN_POINT('Ctrl Pts',(-50.1637036296667,58.7900916492096,173.229373436177));
#44426=CARTESIAN_POINT('Ctrl Pts',(-50.1566568626439,58.7986163344981,173.225789962875));
#44427=CARTESIAN_POINT('Ctrl Pts',(-50.1292096274332,58.8318200776407,173.211832294876));
#44428=CARTESIAN_POINT('Ctrl Pts',(-50.1019214691877,58.8647828422331,173.197227737558));
#44429=CARTESIAN_POINT('Ctrl Pts',(-50.0747632184024,58.8974130720074,173.181821868794));
#44430=CARTESIAN_POINT('Ctrl Pts',(-50.0486290122832,58.9288129275201,173.166996902603));
#44431=CARTESIAN_POINT('Ctrl Pts',(-50.0226148881682,58.9599046602197,173.15142954025));
#44432=CARTESIAN_POINT('Ctrl Pts',(-49.9967338141118,58.990619871463,173.134958085307));
#44433=CARTESIAN_POINT('Ctrl Pts',(-49.9715189975838,59.0205443797903,173.11891065569));
#44434=CARTESIAN_POINT('Ctrl Pts',(-49.9464301568035,59.0501112772456,173.10200475355));
#44435=CARTESIAN_POINT('Ctrl Pts',(-49.9215209152558,59.0792731406212,173.084072502622));
#44436=CARTESIAN_POINT('Ctrl Pts',(-49.8976983277173,59.10716283135,173.066922537752));
#44437=CARTESIAN_POINT('Ctrl Pts',(-49.8740398428972,59.1346818980189,173.0488334264));
#44438=CARTESIAN_POINT('Ctrl Pts',(-49.8506341911061,59.1618061936532,173.029646546259));
#44439=CARTESIAN_POINT('Ctrl Pts',(-49.8334276260605,59.1817465038532,173.015541393191));
#44440=CARTESIAN_POINT('Ctrl Pts',(-49.8163585066683,59.2014737900901,173.000842678105));
#44441=CARTESIAN_POINT('Ctrl Pts',(-49.7994785223376,59.2209856988867,172.985485069079));
#44442=CARTESIAN_POINT('Origin',(-36.5934363437889,54.2142642791517,179.485485069079));
#44443=CARTESIAN_POINT('',(-51.5230382845183,55.5506847976022,178.485485069079));
#44444=CARTESIAN_POINT('',(-51.2438457370575,57.3835762739533,178.485485069079));
#44445=CARTESIAN_POINT('Origin',(-36.5934363437889,54.2142642791517,178.485485069079));
#44446=CARTESIAN_POINT('',(-50.6604618554941,55.4734714302896,178.985485069079));
#44447=CARTESIAN_POINT('Origin',(-51.5230382845183,55.5506847976022,179.485485069079));
#44448=CARTESIAN_POINT('',(-49.7994785223364,59.2209856988899,178.985485069079));
#44449=CARTESIAN_POINT('Origin',(-36.5934363437889,54.2142642791517,178.985485069079));
#44450=CARTESIAN_POINT('Ctrl Pts',(-49.7994785223364,59.2209856988899,178.985485069079));
#44451=CARTESIAN_POINT('Ctrl Pts',(-49.9141823963008,59.0883972151807,178.881126130375));
#44452=CARTESIAN_POINT('Ctrl Pts',(-50.034723824992,58.9461165755505,178.807211858702));
#44453=CARTESIAN_POINT('Ctrl Pts',(-50.2779781597796,58.6518561196932,178.683459642416));
#44454=CARTESIAN_POINT('Ctrl Pts',(-50.4016974430789,58.4986739453797,178.635233133972));
#44455=CARTESIAN_POINT('Ctrl Pts',(-50.7690434736068,58.0324067380221,178.521551735829));
#44456=CARTESIAN_POINT('Ctrl Pts',(-51.0091426506735,57.7124989205671,178.485485069079));
#44457=CARTESIAN_POINT('Ctrl Pts',(-51.2438457370575,57.3835762739533,178.485485069079));
#44458=CARTESIAN_POINT('Origin',(54.4964231308939,46.060372587574,178.485485069079));
#44459=CARTESIAN_POINT('',(-44.6376627105729,59.1917481581946,179.985485069079));
#44460=CARTESIAN_POINT('',(-44.3552179209134,61.1717279657211,179.985485069079));
#44461=CARTESIAN_POINT('Origin',(54.4964231308939,46.060372587574,179.985485069079));
#44462=CARTESIAN_POINT('',(-44.6376627105729,59.1917481581946,171.985485069079));
#44463=CARTESIAN_POINT('',(-44.6376627105729,59.1917481581946,178.485485069079));
#44464=CARTESIAN_POINT('',(-44.3552179209134,61.1717279657211,171.985485069079));
#44465=CARTESIAN_POINT('Origin',(54.4964231308939,46.060372587574,171.985485069079));
#44466=CARTESIAN_POINT('',(-44.3552179209134,61.1717279657211,178.485485069079));
#44467=CARTESIAN_POINT('Origin',(-69.9391102914966,14.1820463536532,178.485485069079));
#44468=CARTESIAN_POINT('',(-73.6640989790157,19.3863195284447,178.485485069079));
#44469=CARTESIAN_POINT('',(-67.3821392712318,8.31502843979556,178.485485069079));
#44470=CARTESIAN_POINT('Origin',(54.4964231308939,46.060372587574,178.485485069079));
#44471=CARTESIAN_POINT('',(-45.4928245268247,44.5939644440383,171.985485069079));
#44472=CARTESIAN_POINT('',(-45.4934286935833,44.6357561061623,171.985485069079));
#44473=CARTESIAN_POINT('Origin',(54.4964231308939,46.060372587574,171.985485069079));
#44474=CARTESIAN_POINT('',(-45.4934286935833,44.6357561061623,179.985485069079));
#44475=CARTESIAN_POINT('',(-45.4934286935833,44.6357561061623,178.485485069079));
#44476=CARTESIAN_POINT('',(-45.4928245268247,44.5939644440384,179.985485069079));
#44477=CARTESIAN_POINT('Origin',(54.4964231308939,46.060372587574,179.985485069079));
#44478=CARTESIAN_POINT('',(-45.4928245268247,44.5939644440383,178.485485069079));
#44479=CARTESIAN_POINT('Origin',(54.4964231308939,46.060372587574,178.485485069079));
#44480=CARTESIAN_POINT('',(-45.0253923549998,36.292658300611,179.985485069079));
#44481=CARTESIAN_POINT('',(-45.451589062978,42.836266743522,179.985485069079));
#44482=CARTESIAN_POINT('Origin',(54.4964231308939,46.060372587574,179.985485069079));
#44483=CARTESIAN_POINT('',(-44.9520576904499,35.5723002038223,178.735485069079));
#44484=CARTESIAN_POINT('Origin',(330.563412065017,138.023170518389,142.559792216127));
#44485=CARTESIAN_POINT('',(-44.8071649770098,34.2791422233116,177.985485069079));
#44486=CARTESIAN_POINT('Ctrl Pts',(-44.9520576904499,35.5723002038223,178.735485069079));
#44487=CARTESIAN_POINT('Ctrl Pts',(-44.9499126757554,35.5519610561786,178.70015248117));
#44488=CARTESIAN_POINT('Ctrl Pts',(-44.9476202963097,35.5302873872292,178.665928645697));
#44489=CARTESIAN_POINT('Ctrl Pts',(-44.9451866758168,35.5073596552394,178.632760823269));
#44490=CARTESIAN_POINT('Ctrl Pts',(-44.9426873271152,35.4838126817709,178.598697190849));
#44491=CARTESIAN_POINT('Ctrl Pts',(-44.9400389751137,35.4589425734026,178.565746780528));
#44492=CARTESIAN_POINT('Ctrl Pts',(-44.9372429317707,35.4327874712696,178.533876632703));
#44493=CARTESIAN_POINT('Ctrl Pts',(-44.9353113405311,35.4147187362919,178.511859771449));
#44494=CARTESIAN_POINT('Ctrl Pts',(-44.9333091525668,35.3960357141058,178.490358963154));
#44495=CARTESIAN_POINT('Ctrl Pts',(-44.9312354927774,35.3767394852785,178.469372146658));
#44496=CARTESIAN_POINT('Ctrl Pts',(-44.9298545854397,35.3638895934528,178.455396445803));
#44497=CARTESIAN_POINT('Ctrl Pts',(-44.9284419618016,35.3507675824538,178.44164883223));
#44498=CARTESIAN_POINT('Ctrl Pts',(-44.9269971286527,35.3373718075001,178.428130798924));
#44499=CARTESIAN_POINT('Ctrl Pts',(-44.9253730263247,35.3223139378043,178.412935501545));
#44500=CARTESIAN_POINT('Ctrl Pts',(-44.9237088282253,35.3069157690946,178.398036553842));
#44501=CARTESIAN_POINT('Ctrl Pts',(-44.9220065207789,35.2911999094899,178.383460539299));
#44502=CARTESIAN_POINT('Ctrl Pts',(-44.918400844352,35.2579119716227,178.352586919996));
#44503=CARTESIAN_POINT('Ctrl Pts',(-44.9146235494019,35.2231928856741,178.323158754952));
#44504=CARTESIAN_POINT('Ctrl Pts',(-44.9106921304939,35.1872437159977,178.295385385406));
#44505=CARTESIAN_POINT('Ctrl Pts',(-44.9063770122815,35.1477859730238,178.264901385722));
#44506=CARTESIAN_POINT('Ctrl Pts',(-44.9018762872234,35.1068472166844,178.236413498132));
#44507=CARTESIAN_POINT('Ctrl Pts',(-44.8972185382424,35.0647396054761,178.210178749903));
#44508=CARTESIAN_POINT('Ctrl Pts',(-44.8957587852626,35.0515429494971,178.201956698423));
#44509=CARTESIAN_POINT('Ctrl Pts',(-44.8942836344116,35.0382316780069,178.193955623614));
#44510=CARTESIAN_POINT('Ctrl Pts',(-44.8927940303359,35.0248158702409,178.18618248533));
#44511=CARTESIAN_POINT('Ctrl Pts',(-44.8927687237777,35.0245879520142,178.186050429182));
#44512=CARTESIAN_POINT('Ctrl Pts',(-44.8927434126584,35.0243600001049,178.185918436739));
#44513=CARTESIAN_POINT('Ctrl Pts',(-44.8927180969803,35.0241320145436,178.18578650803));
#44514=CARTESIAN_POINT('Ctrl Pts',(-44.8821478779092,34.9289397260715,178.130701459469));
#44515=CARTESIAN_POINT('Ctrl Pts',(-44.8705984589575,34.8262343682704,178.085693995916));
#44516=CARTESIAN_POINT('Ctrl Pts',(-44.8585873663329,34.7209813356256,178.052814110577));
#44517=CARTESIAN_POINT('Ctrl Pts',(-44.8564349967444,34.702120151748,178.046922084973));
#44518=CARTESIAN_POINT('Ctrl Pts',(-44.8542678150691,34.6831772657595,178.04141942219));
#44519=CARTESIAN_POINT('Ctrl Pts',(-44.8520888140828,34.6641813681723,178.036317803549));
#44520=CARTESIAN_POINT('Ctrl Pts',(-44.8520700304822,34.6640176181987,178.036273826163));
#44521=CARTESIAN_POINT('Ctrl Pts',(-44.8520512460038,34.66385386429,178.036229878571));
#44522=CARTESIAN_POINT('Ctrl Pts',(-44.8520324606494,34.6636901064642,178.036185960779));
#44523=CARTESIAN_POINT('Ctrl Pts',(-44.8376820744672,34.5385932893174,178.002636566354));
#44524=CARTESIAN_POINT('Ctrl Pts',(-44.8227435745058,34.4104536891947,177.985485079909));
#44525=CARTESIAN_POINT('Ctrl Pts',(-44.8071649770098,34.2791422233116,177.985485069079));
#44526=CARTESIAN_POINT('',(-42.790908491833,22.9265206443813,177.985485069079));
#44527=CARTESIAN_POINT('Origin',(54.4964231308939,46.060372587574,177.985485069079));
#44528=CARTESIAN_POINT('',(-42.790908491833,22.9265206443813,173.985485069079));
#44529=CARTESIAN_POINT('',(-42.790908491833,22.9265206443813,178.485485069079));
#44530=CARTESIAN_POINT('',(-44.8071649770098,34.2791422233116,173.985485069079));
#44531=CARTESIAN_POINT('Origin',(54.4964231308939,46.060372587574,173.985485069079));
#44532=CARTESIAN_POINT('',(-44.9520576904499,35.5723002038223,173.235485069079));
#44533=CARTESIAN_POINT('Ctrl Pts',(-44.8071649770098,34.2791422233116,173.985485069079));
#44534=CARTESIAN_POINT('Ctrl Pts',(-44.8119869746675,34.3197866767732,173.985485066031));
#44535=CARTESIAN_POINT('Ctrl Pts',(-44.8167478717134,34.3601484678123,173.98376136592));
#44536=CARTESIAN_POINT('Ctrl Pts',(-44.8214510473818,34.4002312816899,173.980411411577));
#44537=CARTESIAN_POINT('Ctrl Pts',(-44.8262327788271,34.4409835871633,173.977005503919));
#44538=CARTESIAN_POINT('Ctrl Pts',(-44.8309549221569,34.4814482509048,173.971918425354));
#44539=CARTESIAN_POINT('Ctrl Pts',(-44.8356207182126,34.5216340913495,173.96519866512));
#44540=CARTESIAN_POINT('Ctrl Pts',(-44.840324783733,34.5621495412727,173.958423788541));
#44541=CARTESIAN_POINT('Ctrl Pts',(-44.8449716560963,34.6023823536389,173.949989180473));
#44542=CARTESIAN_POINT('Ctrl Pts',(-44.8495631331995,34.6423350907661,173.939892529448));
#44543=CARTESIAN_POINT('Ctrl Pts',(-44.8504282877738,34.6498632331274,173.937990055881));
#44544=CARTESIAN_POINT('Ctrl Pts',(-44.8512914691809,34.6573813936389,173.936028428795));
#44545=CARTESIAN_POINT('Ctrl Pts',(-44.8521526796834,34.6648895283819,173.934007434543));
#44546=CARTESIAN_POINT('Ctrl Pts',(-44.8577166639521,34.7133969995249,173.920950487154));
#44547=CARTESIAN_POINT('Ctrl Pts',(-44.863192299931,34.7614335526644,173.905424660321));
#44548=CARTESIAN_POINT('Ctrl Pts',(-44.868534832102,34.8085874640509,173.887514455428));
#44549=CARTESIAN_POINT('Ctrl Pts',(-44.873830087861,34.8553241074322,173.869762739094));
#44550=CARTESIAN_POINT('Ctrl Pts',(-44.878994490974,34.9011927505699,173.849668972682));
#44551=CARTESIAN_POINT('Ctrl Pts',(-44.8839868989568,34.9458079142411,173.827363567394));
#44552=CARTESIAN_POINT('Ctrl Pts',(-44.8869886981608,34.9726337993163,173.813951933556));
#44553=CARTESIAN_POINT('Ctrl Pts',(-44.8899283696412,34.9990068755471,173.799741635272));
#44554=CARTESIAN_POINT('Ctrl Pts',(-44.8927976120671,35.0248481275786,173.784768767412));
#44555=CARTESIAN_POINT('Ctrl Pts',(-44.8928230557535,35.0250772809982,173.784635991962));
#44556=CARTESIAN_POINT('Ctrl Pts',(-44.8928484950895,35.0253064026888,173.784503151269));
#44557=CARTESIAN_POINT('Ctrl Pts',(-44.8928739300679,35.0255354925777,173.784370245394));
#44558=CARTESIAN_POINT('Ctrl Pts',(-44.9042559455637,35.1280519808853,173.724895584076));
#44559=CARTESIAN_POINT('Ctrl Pts',(-44.9148445610927,35.2249133976643,173.651948159166));
#44560=CARTESIAN_POINT('Ctrl Pts',(-44.9241349512787,35.3108325653701,173.569559139244));
#44561=CARTESIAN_POINT('Ctrl Pts',(-44.9250117892063,35.3189417172401,173.561783166864));
#44562=CARTESIAN_POINT('Ctrl Pts',(-44.925877066944,35.3269534368476,173.55392308958));
#44563=CARTESIAN_POINT('Ctrl Pts',(-44.9267303628307,35.3348633053383,173.545982294554));
#44564=CARTESIAN_POINT('Ctrl Pts',(-44.9267467660432,35.3350153595733,173.545829645807));
#44565=CARTESIAN_POINT('Ctrl Pts',(-44.9267631651733,35.3351673791874,173.54567696713));
#44566=CARTESIAN_POINT('Ctrl Pts',(-44.9267795602214,35.3353193641777,173.545524258522));
#44567=CARTESIAN_POINT('Ctrl Pts',(-44.9366852808817,35.427147143843,173.453259276234));
#44568=CARTESIAN_POINT('Ctrl Pts',(-44.9451008609219,35.5063351625277,173.350077657882));
#44569=CARTESIAN_POINT('Ctrl Pts',(-44.9520576904499,35.5723002038223,173.235485069079));
#44570=CARTESIAN_POINT('',(-45.0253923549998,36.2926583006112,171.985485069079));
#44571=CARTESIAN_POINT('Origin',(330.563412025084,138.023170571188,209.41117795471));
#44572=CARTESIAN_POINT('',(-45.451589062978,42.836266743522,171.985485069079));
#44573=CARTESIAN_POINT('Origin',(54.4964231308939,46.060372587574,171.985485069079));
#44574=CARTESIAN_POINT('',(-45.451589062978,42.836266743522,178.485485069079));
#44575=CARTESIAN_POINT('Origin',(54.4964231308939,46.060372587574,178.485485069079));
#44576=CARTESIAN_POINT('',(-45.5029364314847,46.4182651889755,171.985485069079));
#44577=CARTESIAN_POINT('',(-45.5028724868992,46.4357070320802,171.985485069079));
#44578=CARTESIAN_POINT('Origin',(54.4964231308939,46.060372587574,171.985485069079));
#44579=CARTESIAN_POINT('',(-45.5028724868992,46.4357070320802,179.985485069079));
#44580=CARTESIAN_POINT('',(-45.5028724868992,46.4357070320801,178.485485069079));
#44581=CARTESIAN_POINT('',(-45.5029364314846,46.4182651889755,179.985485069079));
#44582=CARTESIAN_POINT('Origin',(54.4964231308939,46.060372587574,179.985485069079));
#44583=CARTESIAN_POINT('',(-45.5029364314846,46.4182651889755,178.485485069079));
#44584=CARTESIAN_POINT('Origin',(-55.2932569457149,10.3110887801052,178.485485069079));
#44585=CARTESIAN_POINT('',(-56.491837111464,13.061253427226,173.985485069079));
#44586=CARTESIAN_POINT('',(-56.491837111464,13.061253427226,174.785485069079));
#44587=CARTESIAN_POINT('',(-56.491837111464,13.061253427226,178.485485069079));
#44588=CARTESIAN_POINT('',(-52.503810530151,11.4151669905134,173.985485069079));
#44589=CARTESIAN_POINT('Origin',(-55.2932569457149,10.3110887801052,173.985485069079));
#44590=CARTESIAN_POINT('',(-52.503810530151,11.4151669905134,174.785485069079));
#44591=CARTESIAN_POINT('',(-52.503810530151,11.4151669905134,178.485485069079));
#44592=CARTESIAN_POINT('Origin',(-55.2932569457149,10.3110887801052,174.785485069079));
#44593=CARTESIAN_POINT('Origin',(-69.9391102914966,14.1820463536532,178.485485069079));
#44594=CARTESIAN_POINT('',(-36.2883138077383,14.3227057076466,178.485485069079));
#44595=CARTESIAN_POINT('',(-43.2773451499467,22.8108513846653,178.485485069079));
#44596=CARTESIAN_POINT('Origin',(-31.1164286971058,25.7025828775644,178.485485069079));
#44597=CARTESIAN_POINT('',(-45.3036829175493,34.2202360714903,178.485485069079));
#44598=CARTESIAN_POINT('Origin',(54.4964231308939,46.060372587574,178.485485069079));
#44599=CARTESIAN_POINT('',(-51.7918181085456,40.3156359630969,178.485485069079));
#44600=CARTESIAN_POINT('Origin',(-45.3578332448047,40.663384199939,178.485485069079));
#44601=CARTESIAN_POINT('Origin',(54.4964231308939,46.060372587574,178.485485069079));
#44602=CARTESIAN_POINT('',(-58.9792278552929,42.2495403530246,178.485485069079));
#44603=CARTESIAN_POINT('Origin',(-31.8232466514532,37.9133340783293,178.485485069079));
#44604=CARTESIAN_POINT('Origin',(-94.0351308638859,47.8471884530858,178.485485069079));
#44605=CARTESIAN_POINT('',(-56.6916004724222,13.5196142017461,178.485485069079));
#44606=CARTESIAN_POINT('',(-67.58190263219,8.77338921431569,178.485485069079));
#44607=CARTESIAN_POINT('',(-52.0389027942237,11.5991800255814,178.485485069079));
#44608=CARTESIAN_POINT('Origin',(-55.2932569457149,10.3110887801052,178.485485069079));
#44609=CARTESIAN_POINT('',(-39.8623336503921,1.96564996953346,178.485485069079));
#44610=CARTESIAN_POINT('Origin',(-37.6267629804773,17.3035841126903,178.485485069079));
#44611=CARTESIAN_POINT('Origin',(-38.9776940652673,8.40516957928931,178.485485069079));
#44612=CARTESIAN_POINT('Origin',(-69.9391102914966,14.1820463536532,173.485485069079));
#44613=CARTESIAN_POINT('',(-43.2773451499467,22.8108513846653,173.485485069079));
#44614=CARTESIAN_POINT('',(-36.2883138077383,14.3227057076466,173.485485069079));
#44615=CARTESIAN_POINT('Origin',(-31.1164286971058,25.7025828775644,173.485485069079));
#44616=CARTESIAN_POINT('',(-39.8623336503919,1.96564996953342,173.485485069079));
#44617=CARTESIAN_POINT('Origin',(-38.9776940652673,8.40516957928931,173.485485069079));
#44618=CARTESIAN_POINT('',(-52.0389027942237,11.5991800255814,173.485485069079));
#44619=CARTESIAN_POINT('Origin',(-37.6267629804773,17.3035841126903,173.485485069079));
#44620=CARTESIAN_POINT('',(-56.6916004724222,13.5196142017461,173.485485069079));
#44621=CARTESIAN_POINT('Origin',(-55.2932569457149,10.3110887801052,173.485485069079));
#44622=CARTESIAN_POINT('',(-67.58190263219,8.77338921431569,173.485485069079));
#44623=CARTESIAN_POINT('',(-58.9792278552929,42.2495403530246,173.485485069079));
#44624=CARTESIAN_POINT('Origin',(-94.0351308638859,47.8471884530858,173.485485069079));
#44625=CARTESIAN_POINT('Origin',(-31.8232466514532,37.9133340783293,173.485485069079));
#44626=CARTESIAN_POINT('',(-51.7918181085456,40.3156359630969,173.485485069079));
#44627=CARTESIAN_POINT('Origin',(54.4964231308939,46.060372587574,173.485485069079));
#44628=CARTESIAN_POINT('',(-45.3036829175493,34.2202360714903,173.485485069079));
#44629=CARTESIAN_POINT('Origin',(-45.3578332448047,40.663384199939,173.485485069079));
#44630=CARTESIAN_POINT('Origin',(54.4964231308939,46.060372587574,173.485485069079));
#44631=CARTESIAN_POINT('Origin',(-67.3821392712318,8.31502843979556,178.485485069079));
#44632=CARTESIAN_POINT('',(-56.491837111464,13.061253427226,173.985485069079));
#44633=CARTESIAN_POINT('',(-63.4605999891139,10.0241185510634,174.785485069079));
#44634=CARTESIAN_POINT('',(-63.4605999891139,10.0241185510634,174.785485069079));
#44635=CARTESIAN_POINT('',(-63.4605999891139,10.0241185510634,177.185485069079));
#44636=CARTESIAN_POINT('',(-63.4605999891139,10.0241185510634,177.185485069079));
#44637=CARTESIAN_POINT('',(-56.491837111464,13.061253427226,177.185485069079));
#44638=CARTESIAN_POINT('',(-63.4605999891139,10.0241185510634,177.185485069079));
#44639=CARTESIAN_POINT('',(-56.491837111464,13.061253427226,177.985485069079));
#44640=CARTESIAN_POINT('',(-56.491837111464,13.061253427226,178.485485069079));
#44641=CARTESIAN_POINT('',(-67.3821392712318,8.31502843979556,177.985485069079));
#44642=CARTESIAN_POINT('Origin',(-37.6267629804773,17.3035841126903,178.485485069079));
#44643=CARTESIAN_POINT('',(-39.9344488332926,1.47087790039936,173.985485069079));
#44644=CARTESIAN_POINT('Origin',(-37.6267629804773,17.3035841126903,173.985485069079));
#44645=CARTESIAN_POINT('',(-39.9344488332926,1.47087790039936,177.985485069079));
#44646=CARTESIAN_POINT('',(-39.9344488332926,1.47087790039936,178.485485069079));
#44647=CARTESIAN_POINT('',(-52.503810530151,11.4151669905134,177.985485069079));
#44648=CARTESIAN_POINT('Origin',(-37.6267629804773,17.3035841126903,177.985485069079));
#44649=CARTESIAN_POINT('',(-52.503810530151,11.4151669905134,177.185485069079));
#44650=CARTESIAN_POINT('',(-52.503810530151,11.4151669905134,178.485485069079));
#44651=CARTESIAN_POINT('',(-51.1450921368114,8.74468366806501,177.185485069079));
#44652=CARTESIAN_POINT('Origin',(-37.6267629804773,17.3035841126903,177.185485069079));
#44653=CARTESIAN_POINT('',(-51.1450921368114,8.74468366806501,174.785485069079));
#44654=CARTESIAN_POINT('',(-51.1450921368114,8.74468366806501,178.485485069079));
#44655=CARTESIAN_POINT('Origin',(-37.6267629804773,17.3035841126903,174.785485069079));
#44656=CARTESIAN_POINT('Origin',(-38.9776940652673,8.40516957928931,178.485485069079));
#44657=CARTESIAN_POINT('',(-36.081438403313,14.7779007944433,177.985485069079));
#44658=CARTESIAN_POINT('',(-36.081438403313,14.7779007944433,173.985485069079));
#44659=CARTESIAN_POINT('',(-36.081438403313,14.7779007944433,178.485485069079));
#44660=CARTESIAN_POINT('',(-39.9303828492479,1.47030230724454,177.985485069079));
#44661=CARTESIAN_POINT('Origin',(-38.9776940652673,8.40516957928931,177.985485069079));
#44662=CARTESIAN_POINT('',(-39.9303828492479,1.47030230724454,173.985485069079));
#44663=CARTESIAN_POINT('',(-39.9303828492479,1.47030230724454,178.485485069079));
#44664=CARTESIAN_POINT('Origin',(-38.9776940652673,8.40516957928931,173.985485069079));
#44665=CARTESIAN_POINT('Origin',(-31.1164286971058,25.7025828775644,178.485485069079));
#44666=CARTESIAN_POINT('Origin',(-31.1164286971058,25.7025828775644,177.985485069079));
#44667=CARTESIAN_POINT('Origin',(-31.1164286971058,25.7025828775644,173.985485069079));
#44668=CARTESIAN_POINT('Origin',(-46.8813880107404,61.5195277317696,178.485485069079));
#44669=CARTESIAN_POINT('',(-46.8813880107404,61.5195277317696,171.985485069079));
#44670=CARTESIAN_POINT('',(-31.948047029133,59.4635250419104,171.985485069079));
#44671=CARTESIAN_POINT('',(-46.8813880107404,61.5195277317696,179.985485069079));
#44672=CARTESIAN_POINT('',(-46.8813880107404,61.5195277317696,178.485485069079));
#44673=CARTESIAN_POINT('',(-31.948047029133,59.4635250419104,179.985485069079));
#44674=CARTESIAN_POINT('Origin',(-31.8232466514532,37.9133340783293,178.485485069079));
#44675=CARTESIAN_POINT('',(-48.5106524275047,60.3973392500139,172.002119756093));
#44676=CARTESIAN_POINT('Origin',(-31.8232468038171,37.913334302383,123.527223858898));
#44677=CARTESIAN_POINT('',(-49.7140665684645,59.4521029079787,173.235485069079));
#44678=CARTESIAN_POINT('Ctrl Pts',(-48.5106524258229,60.397339249151,172.002119757177));
#44679=CARTESIAN_POINT('Ctrl Pts',(-48.7316538537475,60.2333141799307,172.21440215845));
#44680=CARTESIAN_POINT('Ctrl Pts',(-48.9480214903638,60.0676803472184,172.429976071149));
#44681=CARTESIAN_POINT('Ctrl Pts',(-49.1601443335358,59.9004207148303,172.648442205403));
#44682=CARTESIAN_POINT('Ctrl Pts',(-49.3480302095647,59.7522720190766,172.841946593724));
#44683=CARTESIAN_POINT('Ctrl Pts',(-49.5325856738131,59.6028469932263,173.037720036652));
#44684=CARTESIAN_POINT('Ctrl Pts',(-49.7140665684645,59.4521029079787,173.235485069079));
#44685=CARTESIAN_POINT('',(-51.5969475386142,57.7375806775091,173.985485069079));
#44686=CARTESIAN_POINT('Ctrl Pts',(-49.7140665684645,59.4521029079787,173.235485069079));
#44687=CARTESIAN_POINT('Ctrl Pts',(-49.7702877045322,59.40540375684,173.296750850855));
#44688=CARTESIAN_POINT('Ctrl Pts',(-49.8290566284154,59.3562043812518,173.351977274771));
#44689=CARTESIAN_POINT('Ctrl Pts',(-49.8897735927165,59.3049226058545,173.402403825032));
#44690=CARTESIAN_POINT('Ctrl Pts',(-49.9574087083972,59.2477977338977,173.458576026648));
#44691=CARTESIAN_POINT('Ctrl Pts',(-50.0274613646153,59.1880887736131,173.508791806356));
#44692=CARTESIAN_POINT('Ctrl Pts',(-50.0991284022786,59.1263501189538,173.554708958926));
#44693=CARTESIAN_POINT('Ctrl Pts',(-50.1165153850139,59.1113718394314,173.565848818547));
#44694=CARTESIAN_POINT('Ctrl Pts',(-50.1339974820091,59.0962740044815,173.57673545706));
#44695=CARTESIAN_POINT('Ctrl Pts',(-50.1515633825625,59.0810643724353,173.587392186236));
#44696=CARTESIAN_POINT('Ctrl Pts',(-50.1520299561151,59.0806603844908,173.587675243059));
#44697=CARTESIAN_POINT('Ctrl Pts',(-50.1524965742564,59.0802563304049,173.587958114495));
#44698=CARTESIAN_POINT('Ctrl Pts',(-50.1529632368644,59.0798522102724,173.588240800684));
#44699=CARTESIAN_POINT('Ctrl Pts',(-50.2598834533621,58.9872615220365,173.65300893928));
#44700=CARTESIAN_POINT('Ctrl Pts',(-50.3690847000011,58.8912502411584,173.708028845801));
#44701=CARTESIAN_POINT('Ctrl Pts',(-50.4789853714511,58.7930624806832,173.754884245436));
#44702=CARTESIAN_POINT('Ctrl Pts',(-50.5283832256402,58.748929313787,173.775944682726));
#44703=CARTESIAN_POINT('Ctrl Pts',(-50.5779226519178,58.7043561380883,173.795354969797));
#44704=CARTESIAN_POINT('Ctrl Pts',(-50.6274609387914,58.6594548008981,173.813255995888));
#44705=CARTESIAN_POINT('Ctrl Pts',(-50.6279626824395,58.6590000221371,173.813437304663));
#44706=CARTESIAN_POINT('Ctrl Pts',(-50.6284644410244,58.6585451959672,173.813618467378));
#44707=CARTESIAN_POINT('Ctrl Pts',(-50.6289662145065,58.6580903224183,173.813799484048));
#44708=CARTESIAN_POINT('Ctrl Pts',(-50.7487120446439,58.5495369359429,173.856998242433));
#44709=CARTESIAN_POINT('Ctrl Pts',(-50.8693781916856,58.4382190449704,173.891907000424));
#44710=CARTESIAN_POINT('Ctrl Pts',(-50.9902670073361,58.3246866825487,173.918668263286));
#44711=CARTESIAN_POINT('Ctrl Pts',(-51.1134618427744,58.208988628678,173.945940011766));
#44712=CARTESIAN_POINT('Ctrl Pts',(-51.2368872549444,58.0909912797521,173.964750480356));
#44713=CARTESIAN_POINT('Ctrl Pts',(-51.3598062968599,57.9712894091945,173.975303121585));
#44714=CARTESIAN_POINT('Ctrl Pts',(-51.4391294462271,57.8940423918909,173.982113040727));
#44715=CARTESIAN_POINT('Ctrl Pts',(-51.5182417735722,57.816085767135,173.985485068216));
#44716=CARTESIAN_POINT('Ctrl Pts',(-51.5969475386142,57.7375806775091,173.985485069079));
#44717=CARTESIAN_POINT('',(-59.47297296809,42.32838046711,173.985485069079));
#44718=CARTESIAN_POINT('Origin',(-31.8232466514532,37.9133340783293,173.985485069079));
#44719=CARTESIAN_POINT('',(-59.47297296809,42.32838046711,177.985485069079));
#44720=CARTESIAN_POINT('',(-59.47297296809,42.32838046711,178.485485069079));
#44721=CARTESIAN_POINT('',(-51.5969475386134,57.7375806775099,177.985485069079));
#44722=CARTESIAN_POINT('Origin',(-31.8232466514532,37.9133340783293,177.985485069079));
#44723=CARTESIAN_POINT('',(-49.7140665684619,59.4521029079808,178.735485069082));
#44724=CARTESIAN_POINT('Ctrl Pts',(-51.5969475386134,57.7375806775099,177.985485069079));
#44725=CARTESIAN_POINT('Ctrl Pts',(-51.433703588371,57.9004084060484,177.985485071801));
#44726=CARTESIAN_POINT('Ctrl Pts',(-51.2699997021575,58.0596677833207,177.999692054503));
#44727=CARTESIAN_POINT('Ctrl Pts',(-51.1060428182335,58.2153933063291,178.028948066425));
#44728=CARTESIAN_POINT('Ctrl Pts',(-50.9473469135473,58.3661219745319,178.057265323794));
#44729=CARTESIAN_POINT('Ctrl Pts',(-50.788413804564,58.5135399732425,178.099681112438));
#44730=CARTESIAN_POINT('Ctrl Pts',(-50.6294298361607,58.6576700285617,178.157004738339));
#44731=CARTESIAN_POINT('Ctrl Pts',(-50.6289321865702,58.6581211826229,178.157184172021));
#44732=CARTESIAN_POINT('Ctrl Pts',(-50.6284345366926,58.6585723042698,178.157363751845));
#44733=CARTESIAN_POINT('Ctrl Pts',(-50.6279368865303,58.6590233935062,178.157543477836));
#44734=CARTESIAN_POINT('Ctrl Pts',(-50.5201533201667,58.7567225611635,178.196469433668));
#44735=CARTESIAN_POINT('Ctrl Pts',(-50.4124428574924,58.8527839753199,178.242613327577));
#44736=CARTESIAN_POINT('Ctrl Pts',(-50.3069537754469,58.9455000636963,178.296772170668));
#44737=CARTESIAN_POINT('Ctrl Pts',(-50.2547510309871,58.9913819139786,178.323573430014));
#44738=CARTESIAN_POINT('Ctrl Pts',(-50.2030925436158,59.0364442219574,178.352338018868));
#44739=CARTESIAN_POINT('Ctrl Pts',(-50.1522410770556,59.0804775615926,178.383166052784));
#44740=CARTESIAN_POINT('Ctrl Pts',(-50.151769832075,59.0808856223957,178.383451738866));
#44741=CARTESIAN_POINT('Ctrl Pts',(-50.1512986579747,59.0812935934674,178.383737601257));
#44742=CARTESIAN_POINT('Ctrl Pts',(-50.1508275549506,59.0817014746528,178.384023640042));
#44743=CARTESIAN_POINT('Ctrl Pts',(-50.0801323160474,59.1429094405883,178.426947542415));
#44744=CARTESIAN_POINT('Ctrl Pts',(-50.0105901739914,59.2024832025505,178.473668141392));
#44745=CARTESIAN_POINT('Ctrl Pts',(-49.9429408461552,59.2599050601864,178.52593231009));
#44746=CARTESIAN_POINT('Ctrl Pts',(-49.8833761345708,59.3104645631132,178.571950507672));
#44747=CARTESIAN_POINT('Ctrl Pts',(-49.8252786144112,59.3593558598453,178.622266054504));
#44748=CARTESIAN_POINT('Ctrl Pts',(-49.7691680069517,59.4062115438254,178.678108553083));
#44749=CARTESIAN_POINT('Ctrl Pts',(-49.7505761117354,59.421736878629,178.696611612116));
#44750=CARTESIAN_POINT('Ctrl Pts',(-49.7322025031268,59.4370385956386,178.715721822545));
#44751=CARTESIAN_POINT('Ctrl Pts',(-49.7140665684645,59.4521029079787,178.735485069079));
#44752=CARTESIAN_POINT('',(-48.5106524275049,60.3973392500138,179.968850382066));
#44753=CARTESIAN_POINT('Ctrl Pts',(-49.7140665684619,59.4521029079808,178.735485069082));
#44754=CARTESIAN_POINT('Ctrl Pts',(-49.509174938667,59.622292730814,178.958761463483));
#44755=CARTESIAN_POINT('Ctrl Pts',(-49.3003647583648,59.790802054021,179.179499303694));
#44756=CARTESIAN_POINT('Ctrl Pts',(-49.0872665483285,59.9576897504803,179.397299299844));
#44757=CARTESIAN_POINT('Ctrl Pts',(-48.898516749987,60.1055090073713,179.590213662405));
#44758=CARTESIAN_POINT('Ctrl Pts',(-48.7064024274161,60.2520555382595,179.78082317782));
#44759=CARTESIAN_POINT('Ctrl Pts',(-48.510652425823,60.3973392491509,179.968850380982));
#44760=CARTESIAN_POINT('Origin',(-31.8232463273633,37.9133336074862,228.443747738763));
#44761=CARTESIAN_POINT('Origin',(-94.0351308638859,47.8471884530858,178.485485069079));
#44762=CARTESIAN_POINT('Origin',(-94.0351308638859,47.8471884530858,177.985485069079));
#44763=CARTESIAN_POINT('Origin',(-94.0351308638859,47.8471884530858,173.985485069079));
#44764=CARTESIAN_POINT('Origin',(-38.9776940652673,8.4051695792893,171.985485069079));
#44765=CARTESIAN_POINT('',(-45.5229719821255,35.6661118192205,171.985485119952));
#44766=CARTESIAN_POINT('Ctrl Pts',(-45.0253923549778,36.2926583001986,171.985485069079));
#44767=CARTESIAN_POINT('Ctrl Pts',(-45.0176017947525,36.2132814174925,171.985485069079));
#44768=CARTESIAN_POINT('Ctrl Pts',(-45.0239871095741,36.1325427086669,171.985485069079));
#44769=CARTESIAN_POINT('Ctrl Pts',(-45.0636400627614,35.9874810744531,171.985485069079));
#44770=CARTESIAN_POINT('Ctrl Pts',(-45.0937395261308,35.9226089710175,171.985485069079));
#44771=CARTESIAN_POINT('Ctrl Pts',(-45.1741039151965,35.811784947861,171.985485069079));
#44772=CARTESIAN_POINT('Ctrl Pts',(-45.2225142153187,35.7657141441877,171.985485069079));
#44773=CARTESIAN_POINT('Ctrl Pts',(-45.3170765407724,35.7079918417109,171.985485069079));
#44774=CARTESIAN_POINT('Ctrl Pts',(-45.35816069493,35.6904301269908,171.985485069079));
#44775=CARTESIAN_POINT('Ctrl Pts',(-45.4411069174444,35.6692181889851,171.985485069079));
#44776=CARTESIAN_POINT('Ctrl Pts',(-45.4819542285517,35.6647560993595,171.985485069079));
#44777=CARTESIAN_POINT('Ctrl Pts',(-45.5229716741717,35.666111487147,171.985485069079));
#44778=CARTESIAN_POINT('',(-50.3505460635896,40.3935347805572,171.985485069079));
#44779=CARTESIAN_POINT('Origin',(-45.3578332448047,40.663384199939,171.985485069079));
#44780=CARTESIAN_POINT('',(-50.0854109028112,55.4219958520818,171.985485069079));
#44781=CARTESIAN_POINT('Origin',(54.4964231308939,46.060372587574,171.985485069079));
#44782=CARTESIAN_POINT('',(-48.8396164156005,60.0041865017348,171.985485044813));
#44783=CARTESIAN_POINT('Origin',(-36.5934363437889,54.2142642791517,171.985485069079));
#44784=CARTESIAN_POINT('',(-48.5925895957766,60.3286139604208,171.985485069079));
#44785=CARTESIAN_POINT('Ctrl Pts',(-48.8396208834494,60.0041886143,171.985485069079));
#44786=CARTESIAN_POINT('Ctrl Pts',(-48.8104873581851,60.0658028957206,171.985485069079));
#44787=CARTESIAN_POINT('Ctrl Pts',(-48.7734354054051,60.1243517973398,171.985485071599));
#44788=CARTESIAN_POINT('Ctrl Pts',(-48.6900390743796,60.2323373406952,171.985485071599));
#44789=CARTESIAN_POINT('Ctrl Pts',(-48.6430278708974,60.2826903631409,171.985485069079));
#44790=CARTESIAN_POINT('Ctrl Pts',(-48.5925895957754,60.3286139604194,171.985485069079));
#44791=CARTESIAN_POINT('',(-66.4598969965647,47.8938297558071,171.985485069079));
#44792=CARTESIAN_POINT('',(-45.7483677109949,58.3231663243772,171.985485069079));
#44793=CARTESIAN_POINT('',(-44.6376627105729,59.1917481581946,171.985485069079));
#44794=CARTESIAN_POINT('',(-44.949586852714,57.3017198020218,171.985485069079));
#44795=CARTESIAN_POINT('',(-45.7483677109949,58.3231663243772,171.985485069079));
#44796=CARTESIAN_POINT('',(-45.9329959574027,56.5326845647457,171.985485069079));
#44797=CARTESIAN_POINT('',(-44.8222909569807,57.4012663985631,171.985485069079));
#44798=CARTESIAN_POINT('',(-45.1205026113461,55.4937031042329,171.985485069079));
#44799=CARTESIAN_POINT('',(-45.9329959574027,56.5326845647457,171.985485069079));
#44800=CARTESIAN_POINT('',(-46.0853673634888,54.7391697263481,171.985485069079));
#44801=CARTESIAN_POINT('',(-44.9746623630668,55.6077515601656,171.985485069079));
#44802=CARTESIAN_POINT('',(-45.2594247703932,53.6829899485823,171.985485069079));
#44803=CARTESIAN_POINT('',(-46.0853673634888,54.7391697263481,171.985485069079));
#44804=CARTESIAN_POINT('',(-46.2054325622506,52.9432028923028,171.985485069079));
#44805=CARTESIAN_POINT('',(-45.0947275618286,53.8117847261202,171.985485069079));
#44806=CARTESIAN_POINT('',(-45.3663083202907,51.8701669902924,171.985485069079));
#44807=CARTESIAN_POINT('',(-46.2054325622506,52.9432028923028,171.985485069079));
#44808=CARTESIAN_POINT('',(-46.293152653614,51.1453659401528,171.985485069079));
#44809=CARTESIAN_POINT('',(-45.182447653192,52.0139477739702,171.985485069079));
#44810=CARTESIAN_POINT('',(-45.4411186317038,50.0558215681434,171.985485069079));
#44811=CARTESIAN_POINT('',(-46.293152653614,51.1453659401528,171.985485069079));
#44812=CARTESIAN_POINT('',(-46.3484992170368,49.3462413533434,171.985485069079));
#44813=CARTESIAN_POINT('',(-45.2377942166148,50.2148231871608,171.985485069079));
#44814=CARTESIAN_POINT('',(-45.4838314667458,48.2405415141803,171.985485069079));
#44815=CARTESIAN_POINT('',(-46.3484992170368,49.3462413533434,171.985485069079));
#44816=CARTESIAN_POINT('',(-46.3714543207166,47.5464120325021,171.985485069079));
#44817=CARTESIAN_POINT('',(-45.2607493202947,48.4149938663196,171.985485069079));
#44818=CARTESIAN_POINT('',(-46.3714543207166,47.5464120325021,171.985485069079));
#44819=CARTESIAN_POINT('',(-46.3620105274007,45.7464611065843,171.985485069079));
#44820=CARTESIAN_POINT('',(-45.2513055269787,46.6150429404017,171.985485069079));
#44821=CARTESIAN_POINT('',(-46.3620105274007,45.7464611065843,171.985485069079));
#44822=CARTESIAN_POINT('',(-46.3201708967954,43.9469717439439,171.985485069079));
#44823=CARTESIAN_POINT('',(-45.2094658963734,44.8155535777614,171.985485069079));
#44824=CARTESIAN_POINT('',(-46.3201708967954,43.9469717439439,171.985485069079));
#44825=CARTESIAN_POINT('Origin',(54.4964231308939,46.060372587574,171.985485069079));
#44826=CARTESIAN_POINT('',(-50.927054881572,40.3623752535731,172.985485069079));
#44827=CARTESIAN_POINT('',(-50.3505460635896,40.3935347805572,171.985485069079));
#44828=CARTESIAN_POINT('Origin',(54.4964231308939,46.060372587574,172.985485069079));
#44829=CARTESIAN_POINT('',(-50.0854109028112,55.4219958520819,171.985485069079));
#44830=CARTESIAN_POINT('Origin',(-36.5934363437889,54.2142642791517,171.985485069079));
#44831=CARTESIAN_POINT('Ctrl Pts',(-49.7994785223376,59.2209856988867,172.985485069079));
#44832=CARTESIAN_POINT('Ctrl Pts',(-49.4892805846571,59.4856670319597,172.645618020514));
#44833=CARTESIAN_POINT('Ctrl Pts',(-49.1697658047785,59.7466931532137,172.311831139785));
#44834=CARTESIAN_POINT('Ctrl Pts',(-48.8396130608551,60.0041835729237,171.985486127831));
#44835=CARTESIAN_POINT('Origin',(-66.4598969965647,47.8938297558071,171.985485069079));
#44836=CARTESIAN_POINT('Ctrl Pts',(-48.5925895957742,60.3286139604199,171.985485069075));
#44837=CARTESIAN_POINT('Ctrl Pts',(-48.5801791134111,60.3407485993548,171.990457348712));
#44838=CARTESIAN_POINT('Ctrl Pts',(-48.5668415570095,60.3526167618077,171.994133545212));
#44839=CARTESIAN_POINT('Ctrl Pts',(-48.5394083236438,60.3754624609016,171.99946969614));
#44840=CARTESIAN_POINT('Ctrl Pts',(-48.525119006316,60.3866023176528,172.001168825203));
#44841=CARTESIAN_POINT('Ctrl Pts',(-48.5106524368776,60.3973392472798,172.002119759697));
#44842=CARTESIAN_POINT('Origin',(-45.3578332448047,40.663384199939,171.985485069079));
#44843=CARTESIAN_POINT('',(-45.4569991048231,35.0869155900178,172.985485069079));
#44844=CARTESIAN_POINT('Origin',(488.633838875382,289.196466346075,284.259200636902));
#44845=CARTESIAN_POINT('Origin',(-45.3578332448047,40.663384199939,172.985485069079));
#44846=CARTESIAN_POINT('Origin',(-45.3578332448047,40.663384199939,179.985485069079));
#44847=CARTESIAN_POINT('',(-50.927054881572,40.3623752535731,178.985485069079));
#44848=CARTESIAN_POINT('',(-45.4569991048231,35.0869155900178,178.985485069079));
#44849=CARTESIAN_POINT('Origin',(-45.3578332448047,40.663384199939,178.985485069079));
#44850=CARTESIAN_POINT('',(-45.5229719821697,35.6661118192729,179.985485018174));
#44851=CARTESIAN_POINT('Origin',(488.633838896208,289.196466334528,67.7117695084859));
#44852=CARTESIAN_POINT('',(-50.3505460635896,40.3935347805572,179.985485069079));
#44853=CARTESIAN_POINT('Origin',(-45.3578332448047,40.663384199939,179.985485069079));
#44854=CARTESIAN_POINT('',(-50.3505460635896,40.3935347805572,179.985485069079));
#44855=CARTESIAN_POINT('Origin',(-66.4598969965647,47.8938297558071,179.985485069079));
#44856=CARTESIAN_POINT('',(-48.5925895957765,60.3286139604208,179.985485069079));
#44857=CARTESIAN_POINT('Ctrl Pts',(-48.5106524368779,60.3973392472796,179.968850378462));
#44858=CARTESIAN_POINT('Ctrl Pts',(-48.5251190063152,60.3866023176534,179.969801312955));
#44859=CARTESIAN_POINT('Ctrl Pts',(-48.5394083236435,60.3754624609018,179.971500442019));
#44860=CARTESIAN_POINT('Ctrl Pts',(-48.5668415570078,60.3526167618089,179.976836592946));
#44861=CARTESIAN_POINT('Ctrl Pts',(-48.5801791134102,60.3407485993553,179.980512789447));
#44862=CARTESIAN_POINT('Ctrl Pts',(-48.5925895957738,60.3286139604199,179.985485069084));
#44863=CARTESIAN_POINT('',(-66.4598969965647,47.8938297558071,179.985485069079));
#44864=CARTESIAN_POINT('Origin',(-36.5934363437889,54.2142642791517,179.985485069079));
#44865=CARTESIAN_POINT('',(-48.8396164156006,60.0041865017348,179.985485093346));
#44866=CARTESIAN_POINT('',(-50.0854109028112,55.4219958520818,179.985485069079));
#44867=CARTESIAN_POINT('Origin',(-36.5934363437889,54.2142642791517,179.985485069079));
#44868=CARTESIAN_POINT('Ctrl Pts',(-48.8396130608551,60.0041835729237,179.985484010327));
#44869=CARTESIAN_POINT('Ctrl Pts',(-49.1697658047781,59.7466931532141,179.659138998374));
#44870=CARTESIAN_POINT('Ctrl Pts',(-49.489280584655,59.4856670319615,179.325352117647));
#44871=CARTESIAN_POINT('Ctrl Pts',(-49.7994785223364,59.2209856988899,178.985485069079));
#44872=CARTESIAN_POINT('',(-50.0854109028112,55.4219958520818,179.985485069079));
#44873=CARTESIAN_POINT('Origin',(54.4964231308939,46.060372587574,179.985485069079));
#44874=CARTESIAN_POINT('Origin',(54.4964231308939,46.060372587574,178.985485069079));
#44875=CARTESIAN_POINT('Origin',(54.4964231308939,46.060372587574,179.985485069079));
#44876=CARTESIAN_POINT('Origin',(-38.9776940652673,8.4051695792893,179.985485069079));
#44877=CARTESIAN_POINT('Ctrl Pts',(-45.5229716741763,35.6661114871472,179.985485069079));
#44878=CARTESIAN_POINT('Ctrl Pts',(-45.4821910556965,35.6647639251181,179.985485069079));
#44879=CARTESIAN_POINT('Ctrl Pts',(-45.4415765396099,35.6691667965979,179.985485069079));
#44880=CARTESIAN_POINT('Ctrl Pts',(-45.3590894448663,35.6901192458687,179.985485069079));
#44881=CARTESIAN_POINT('Ctrl Pts',(-45.3182137267096,35.7074699102648,179.985485069079));
#44882=CARTESIAN_POINT('Ctrl Pts',(-45.2237659769383,35.7647003566238,179.985485069079));
#44883=CARTESIAN_POINT('Ctrl Pts',(-45.175266512742,35.8105527807682,179.985485069079));
#44884=CARTESIAN_POINT('Ctrl Pts',(-45.0946358711023,35.9209880541501,179.985485069079));
#44885=CARTESIAN_POINT('Ctrl Pts',(-45.0643644570102,35.9856925299171,179.985485069079));
#44886=CARTESIAN_POINT('Ctrl Pts',(-45.0240949599695,36.1311938017274,179.985485069079));
#44887=CARTESIAN_POINT('Ctrl Pts',(-45.017536669623,36.2126178670405,179.985485069079));
#44888=CARTESIAN_POINT('Ctrl Pts',(-45.0253923549778,36.2926583001987,179.985485069079));
#44889=CARTESIAN_POINT('',(-46.3201708967954,43.9469717439439,179.985485069079));
#44890=CARTESIAN_POINT('',(-44.1642119224607,41.1900243611352,179.985485069079));
#44891=CARTESIAN_POINT('',(-45.2094658963734,44.8155535777614,179.985485069079));
#44892=CARTESIAN_POINT('',(-46.3620105274007,45.7464611065843,179.985485069079));
#44893=CARTESIAN_POINT('',(-44.206051553066,42.9895137237755,179.985485069079));
#44894=CARTESIAN_POINT('',(-45.2513055269787,46.6150429404017,179.985485069079));
#44895=CARTESIAN_POINT('',(-46.3714543207166,47.5464120325021,179.985485069079));
#44896=CARTESIAN_POINT('',(-44.2154953463819,44.7894646496933,179.985485069079));
#44897=CARTESIAN_POINT('',(-45.4838314667458,48.2405415141803,179.985485069079));
#44898=CARTESIAN_POINT('',(-45.2607493202947,48.4149938663196,179.985485069079));
#44899=CARTESIAN_POINT('',(-46.3484992170368,49.3462413533434,179.985485069079));
#44900=CARTESIAN_POINT('',(-44.1925402427021,46.5892939705346,179.985485069079));
#44901=CARTESIAN_POINT('',(-45.4411186317038,50.0558215681434,179.985485069079));
#44902=CARTESIAN_POINT('',(-45.2377942166148,50.2148231871608,179.985485069079));
#44903=CARTESIAN_POINT('',(-46.293152653614,51.1453659401528,179.985485069079));
#44904=CARTESIAN_POINT('',(-44.1371936792793,48.388418557344,179.985485069079));
#44905=CARTESIAN_POINT('',(-45.3663083202907,51.8701669902924,179.985485069079));
#44906=CARTESIAN_POINT('',(-45.182447653192,52.0139477739702,179.985485069079));
#44907=CARTESIAN_POINT('',(-46.2054325622506,52.9432028923028,179.985485069079));
#44908=CARTESIAN_POINT('',(-44.0494735879158,50.186255509494,179.985485069079));
#44909=CARTESIAN_POINT('',(-45.2594247703932,53.6829899485823,179.985485069079));
#44910=CARTESIAN_POINT('',(-45.0947275618286,53.8117847261202,179.985485069079));
#44911=CARTESIAN_POINT('',(-46.0853673634888,54.7391697263481,179.985485069079));
#44912=CARTESIAN_POINT('',(-43.9294083891541,51.9822223435394,179.985485069079));
#44913=CARTESIAN_POINT('',(-45.1205026113461,55.4937031042329,179.985485069079));
#44914=CARTESIAN_POINT('',(-44.9746623630668,55.6077515601656,179.985485069079));
#44915=CARTESIAN_POINT('',(-45.9329959574027,56.5326845647457,179.985485069079));
#44916=CARTESIAN_POINT('',(-43.777036983068,53.7757371819369,179.985485069079));
#44917=CARTESIAN_POINT('',(-44.949586852714,57.3017198020218,179.985485069079));
#44918=CARTESIAN_POINT('',(-44.8222909569807,57.4012663985631,179.985485069079));
#44919=CARTESIAN_POINT('',(-45.7483677109949,58.3231663243772,179.985485069079));
#44920=CARTESIAN_POINT('',(-43.5924087366602,55.5662189415684,179.985485069079));
#44921=CARTESIAN_POINT('',(-65.7700217936225,42.6660431345655,179.985485069079));
#44922=CARTESIAN_POINT('Ctrl Pts',(-48.5925895957752,60.3286139604194,179.985485069079));
#44923=CARTESIAN_POINT('Ctrl Pts',(-48.6430370917591,60.2826819676288,179.985485069079));
#44924=CARTESIAN_POINT('Ctrl Pts',(-48.6900563305759,60.232318868423,179.985485066651));
#44925=CARTESIAN_POINT('Ctrl Pts',(-48.7734488840562,60.1243304643096,179.985485066651));
#44926=CARTESIAN_POINT('Ctrl Pts',(-48.8104926495586,60.0657917050398,179.985485069079));
#44927=CARTESIAN_POINT('Ctrl Pts',(-48.8396208834495,60.0041886143001,179.985485069079));
#44928=CARTESIAN_POINT('Origin',(-45.3578332448047,40.663384199939,179.485485069079));
#44929=CARTESIAN_POINT('Ctrl Pts',(-45.3036829175493,34.2202360714903,178.485485069079));
#44930=CARTESIAN_POINT('Ctrl Pts',(-45.3189505131708,34.3080655568667,178.485485069079));
#44931=CARTESIAN_POINT('Ctrl Pts',(-45.3338848762283,34.3938033049738,178.496890676795));
#44932=CARTESIAN_POINT('Ctrl Pts',(-45.3485335977834,34.4775333459783,178.519211521199));
#44933=CARTESIAN_POINT('Ctrl Pts',(-45.3485497210739,34.4776255044486,178.519236088903));
#44934=CARTESIAN_POINT('Ctrl Pts',(-45.3485658440143,34.4777176604645,178.519260669829));
#44935=CARTESIAN_POINT('Ctrl Pts',(-45.348581966605,34.4778098140261,178.519285263975));
#44936=CARTESIAN_POINT('Ctrl Pts',(-45.3614851957113,34.5515621375495,178.53896844682));
#44937=CARTESIAN_POINT('Ctrl Pts',(-45.3742367759305,34.6241378461091,178.56762577006));
#44938=CARTESIAN_POINT('Ctrl Pts',(-45.3862037841395,34.6918764218863,178.603791729928));
#44939=CARTESIAN_POINT('Ctrl Pts',(-45.387807086225,34.7009518230151,178.608637131374));
#44940=CARTESIAN_POINT('Ctrl Pts',(-45.3893962981546,34.7099403541399,178.613617373854));
#44941=CARTESIAN_POINT('Ctrl Pts',(-45.3909698892282,34.7188331600865,178.618728986713));
#44942=CARTESIAN_POINT('Ctrl Pts',(-45.3909996250014,34.719001205308,178.618825579635));
#44943=CARTESIAN_POINT('Ctrl Pts',(-45.3910293556473,34.7191692188888,178.61892222093));
#44944=CARTESIAN_POINT('Ctrl Pts',(-45.3910590811527,34.7193372007523,178.61901891057));
#44945=CARTESIAN_POINT('Ctrl Pts',(-45.3968750896393,34.7522040580152,178.637936932599));
#44946=CARTESIAN_POINT('Ctrl Pts',(-45.4025476904675,34.7841474493449,178.658893238736));
#44947=CARTESIAN_POINT('Ctrl Pts',(-45.4080183431112,34.8148573132726,178.681656749639));
#44948=CARTESIAN_POINT('Ctrl Pts',(-45.4135433861197,34.8458725010455,178.704646580094));
#44949=CARTESIAN_POINT('Ctrl Pts',(-45.4188622767047,34.8756286399688,178.729479042991));
#44950=CARTESIAN_POINT('Ctrl Pts',(-45.4239193913347,34.903835066337,178.755872459173));
#44951=CARTESIAN_POINT('Ctrl Pts',(-45.4253049650645,34.9115632050574,178.763103860234));
#44952=CARTESIAN_POINT('Ctrl Pts',(-45.4266709229058,34.9191752174847,178.770452222341));
#44953=CARTESIAN_POINT('Ctrl Pts',(-45.4280162071684,34.9266656301276,178.777911297277));
#44954=CARTESIAN_POINT('Ctrl Pts',(-45.431900150492,34.9482910508554,178.799446243539));
#44955=CARTESIAN_POINT('Ctrl Pts',(-45.4356071123145,34.9688770623761,178.821871912933));
#44956=CARTESIAN_POINT('Ctrl Pts',(-45.4391361091639,34.9884275421567,178.845188937286));
#44957=CARTESIAN_POINT('Ctrl Pts',(-45.4425882966433,35.0075525015699,178.867998461624));
#44958=CARTESIAN_POINT('Ctrl Pts',(-45.4458702772851,35.0256869893978,178.891661629521));
#44959=CARTESIAN_POINT('Ctrl Pts',(-45.4489746253575,35.042796910032,178.916209181352));
#44960=CARTESIAN_POINT('Ctrl Pts',(-45.4518004907941,35.0583719461472,178.938554638967));
#44961=CARTESIAN_POINT('Ctrl Pts',(-45.4544791600941,35.0730979247513,178.961633558394));
#44962=CARTESIAN_POINT('Ctrl Pts',(-45.4569991048231,35.0869155900178,178.985485069079));
#44963=CARTESIAN_POINT('Origin',(-51.7918181085456,40.3156359630969,179.485485069079));
#44964=CARTESIAN_POINT('Origin',(54.4964231308939,46.060372587574,179.485485069079));
#44965=CARTESIAN_POINT('Origin',(-45.3578332448047,40.663384199939,172.485485069079));
#44966=CARTESIAN_POINT('Ctrl Pts',(-45.4569991048231,35.0869155900178,172.985485069079));
#44967=CARTESIAN_POINT('Ctrl Pts',(-45.4494550799535,35.0455492823621,173.056889963465));
#44968=CARTESIAN_POINT('Ctrl Pts',(-45.4405646313053,34.9965213246108,173.121515548973));
#44969=CARTESIAN_POINT('Ctrl Pts',(-45.4304424047398,34.9402282867916,173.179712320665));
#44970=CARTESIAN_POINT('Ctrl Pts',(-45.4296958966764,34.9360767094311,173.184004297243));
#44971=CARTESIAN_POINT('Ctrl Pts',(-45.4289426856633,34.9318855998601,173.188261292746));
#44972=CARTESIAN_POINT('Ctrl Pts',(-45.4281828161243,34.9276551088421,173.192483440716));
#44973=CARTESIAN_POINT('Ctrl Pts',(-45.4281583546134,34.9275189220408,173.192619358941));
#44974=CARTESIAN_POINT('Ctrl Pts',(-45.4281338855781,34.9273826908262,173.192755241168));
#44975=CARTESIAN_POINT('Ctrl Pts',(-45.4281094090274,34.9272464152488,173.192891087362));
#44976=CARTESIAN_POINT('Ctrl Pts',(-45.4181985665645,34.8720668355002,173.247896804654));
#44977=CARTESIAN_POINT('Ctrl Pts',(-45.4070570723305,34.8096241895739,173.296989238882));
#44978=CARTESIAN_POINT('Ctrl Pts',(-45.3952940807049,34.7432514620707,173.337731815262));
#44979=CARTESIAN_POINT('Ctrl Pts',(-45.3939189104418,34.7354920583365,173.342494887554));
#44980=CARTESIAN_POINT('Ctrl Pts',(-45.3925352362935,34.7276788857477,173.347143832958));
#44981=CARTESIAN_POINT('Ctrl Pts',(-45.391144024528,34.71981722941,173.351674748709));
#44982=CARTESIAN_POINT('Ctrl Pts',(-45.391113929105,34.7196471619343,173.351772763857));
#44983=CARTESIAN_POINT('Ctrl Pts',(-45.3910838287156,34.7194770634957,173.351870728113));
#44984=CARTESIAN_POINT('Ctrl Pts',(-45.391053723366,34.7193069341307,173.351968641468));
#44985=CARTESIAN_POINT('Ctrl Pts',(-45.3853123614024,34.686861728367,173.370641602265));
#44986=CARTESIAN_POINT('Ctrl Pts',(-45.3793724983653,34.653189475525,173.387517101079));
#44987=CARTESIAN_POINT('Ctrl Pts',(-45.3732936451112,34.6186406634444,173.402457951648));
#44988=CARTESIAN_POINT('Ctrl Pts',(-45.3671493578082,34.5837199607191,173.41755962866));
#44989=CARTESIAN_POINT('Ctrl Pts',(-45.3608632446221,34.5479047591227,173.430684404547));
#44990=CARTESIAN_POINT('Ctrl Pts',(-45.3545001320436,34.5115782752305,173.44173857501));
#44991=CARTESIAN_POINT('Ctrl Pts',(-45.3525468614839,34.5004272150142,173.445131849208));
#44992=CARTESIAN_POINT('Ctrl Pts',(-45.3505863489167,34.4892280661516,173.448330371619));
#44993=CARTESIAN_POINT('Ctrl Pts',(-45.3486204928608,34.4779920738192,173.451332405848));
#44994=CARTESIAN_POINT('Ctrl Pts',(-45.3434524005459,34.4484534687685,173.459224535072));
#44995=CARTESIAN_POINT('Ctrl Pts',(-45.3382520871963,34.4186872945855,173.465756220107));
#44996=CARTESIAN_POINT('Ctrl Pts',(-45.3330182670165,34.3886927955056,173.470935497225));
#44997=CARTESIAN_POINT('Ctrl Pts',(-45.3278822554434,34.3592588277512,173.476017985026));
#44998=CARTESIAN_POINT('Ctrl Pts',(-45.3227138390104,34.3296041551761,173.479798218183));
#44999=CARTESIAN_POINT('Ctrl Pts',(-45.3175108165138,34.2997211452501,173.482235171309));
#45000=CARTESIAN_POINT('Ctrl Pts',(-45.3129287259598,34.2734043923248,173.484381296933));
#45001=CARTESIAN_POINT('Ctrl Pts',(-45.3083197232477,34.2469100985176,173.485485069079));
#45002=CARTESIAN_POINT('Ctrl Pts',(-45.3036829175493,34.2202360714903,173.485485069079));
#45003=CARTESIAN_POINT('Origin',(-51.7918181085456,40.3156359630969,172.485485069079));
#45004=CARTESIAN_POINT('Origin',(54.4964231308939,46.060372587574,172.485485069079));
#45005=CARTESIAN_POINT('Origin',(-55.2932569457149,10.3110887801052,178.485485069079));
#45006=CARTESIAN_POINT('Origin',(-55.2932569457149,10.3110887801052,177.985485069079));
#45007=CARTESIAN_POINT('Origin',(-55.2932569457149,10.3110887801052,177.185485069079));
#45008=CARTESIAN_POINT('Origin',(-51.5511046852341,5.7956973373016,177.185485069079));
#45009=CARTESIAN_POINT('',(-51.5511046852341,5.7956973373016,174.785485069079));
#45010=CARTESIAN_POINT('',(-51.5511046852341,5.7956973373016,174.785485069079));
#45011=CARTESIAN_POINT('',(-51.5511046852341,5.7956973373016,177.185485069079));
#45012=CARTESIAN_POINT('',(-51.5511046852341,5.7956973373016,177.185485069079));
#45013=CARTESIAN_POINT('',(-51.5511046852341,5.7956973373016,177.185485069079));
#45014=CARTESIAN_POINT('Origin',(-55.2165279528263,6.30034797823479,177.185485069079));
#45015=CARTESIAN_POINT('',(-57.9855837402625,3.84630436695446,177.185485069079));
#45016=CARTESIAN_POINT('',(-63.4605999891139,10.0241185510634,177.185485069079));
#45017=CARTESIAN_POINT('Origin',(-55.2165279528263,6.30034797823479,177.185485069079));
#45018=CARTESIAN_POINT('Origin',(-55.2165279528263,6.30034797823479,174.785485069079));
#45019=CARTESIAN_POINT('',(-57.9855837402625,3.84630436695446,174.785485069079));
#45020=CARTESIAN_POINT('Origin',(-55.2165279528263,6.30034797823479,174.785485069079));
#45021=CARTESIAN_POINT('',(-63.4605999891139,10.0241185510634,174.785485069079));
#45022=CARTESIAN_POINT('Origin',(-55.2165279528263,6.30034797823479,177.185485069079));
#45023=CARTESIAN_POINT('',(-57.9855837402625,3.84630436695446,177.185485069079));
#45024=CARTESIAN_POINT('Origin',(-63.4605999891139,10.0241185510634,177.185485069079));
#45025=CARTESIAN_POINT('Origin',(-43.5924087366602,55.5662189415684,171.985485069079));
#45026=CARTESIAN_POINT('',(-44.949586852714,57.3017198020218,171.985485069079));
#45027=CARTESIAN_POINT('',(-45.7483677109949,58.3231663243772,171.985485069079));
#45028=CARTESIAN_POINT('Origin',(-44.6376627105729,59.1917481581946,171.985485069079));
#45029=CARTESIAN_POINT('Origin',(-44.8222909569807,57.4012663985631,171.985485069079));
#45030=CARTESIAN_POINT('',(-45.9329959574027,56.5326845647457,171.985485069079));
#45031=CARTESIAN_POINT('Origin',(-44.9746623630668,55.6077515601656,171.985485069079));
#45032=CARTESIAN_POINT('',(-46.0853673634888,54.7391697263481,171.985485069079));
#45033=CARTESIAN_POINT('',(-45.1205026113461,55.4937031042329,171.985485069079));
#45034=CARTESIAN_POINT('Origin',(-45.0947275618286,53.8117847261202,171.985485069079));
#45035=CARTESIAN_POINT('',(-46.2054325622506,52.9432028923028,171.985485069079));
#45036=CARTESIAN_POINT('',(-45.2594247703932,53.6829899485823,171.985485069079));
#45037=CARTESIAN_POINT('Origin',(-45.182447653192,52.0139477739702,171.985485069079));
#45038=CARTESIAN_POINT('',(-46.293152653614,51.1453659401528,171.985485069079));
#45039=CARTESIAN_POINT('',(-45.3663083202907,51.8701669902924,171.985485069079));
#45040=CARTESIAN_POINT('Origin',(-45.2377942166148,50.2148231871608,171.985485069079));
#45041=CARTESIAN_POINT('',(-46.3484992170368,49.3462413533434,171.985485069079));
#45042=CARTESIAN_POINT('',(-45.4411186317038,50.0558215681434,171.985485069079));
#45043=CARTESIAN_POINT('Origin',(-45.2607493202947,48.4149938663196,171.985485069079));
#45044=CARTESIAN_POINT('',(-46.3714543207166,47.5464120325021,171.985485069079));
#45045=CARTESIAN_POINT('',(-45.4838314667458,48.2405415141803,171.985485069079));
#45046=CARTESIAN_POINT('Origin',(-44.2154953463819,44.7894646496933,171.985485069079));
#45047=CARTESIAN_POINT('Origin',(-44.1925402427021,46.5892939705346,171.985485069079));
#45048=CARTESIAN_POINT('Origin',(-44.1371936792793,48.388418557344,171.985485069079));
#45049=CARTESIAN_POINT('Origin',(-44.0494735879158,50.186255509494,171.985485069079));
#45050=CARTESIAN_POINT('Origin',(-43.9294083891541,51.9822223435394,171.985485069079));
#45051=CARTESIAN_POINT('Origin',(-43.777036983068,53.7757371819369,171.985485069079));
#45052=CARTESIAN_POINT('Origin',(-45.2094658963734,44.8155535777614,171.985485069079));
#45053=CARTESIAN_POINT('',(-46.3201708967954,43.9469717439439,171.985485069079));
#45054=CARTESIAN_POINT('Origin',(-44.1642119224607,41.1900243611352,171.985485069079));
#45055=CARTESIAN_POINT('Origin',(-44.206051553066,42.9895137237755,171.985485069079));
#45056=CARTESIAN_POINT('',(-46.3620105274007,45.7464611065843,171.985485069079));
#45057=CARTESIAN_POINT('Origin',(-45.2513055269787,46.6150429404017,171.985485069079));
#45058=CARTESIAN_POINT('Origin',(-37.6267629804773,17.3035841126903,173.985485069079));
#45059=CARTESIAN_POINT('Origin',(-39.8623336503921,1.96564996953346,173.985485069079));
#45060=CARTESIAN_POINT('Origin',(-52.0389027942237,11.5991800255814,173.985485069079));
#45061=CARTESIAN_POINT('Origin',(-55.2932569457149,10.3110887801052,173.985485069079));
#45062=CARTESIAN_POINT('Origin',(-56.6916004724222,13.5196142017461,173.985485069079));
#45063=CARTESIAN_POINT('Origin',(-67.58190263219,8.77338921431569,173.985485069079));
#45064=CARTESIAN_POINT('Origin',(-94.0351308638859,47.8471884530858,173.985485069079));
#45065=CARTESIAN_POINT('Origin',(-58.9792278552929,42.2495403530246,173.985485069079));
#45066=CARTESIAN_POINT('Origin',(-31.8232466514532,37.9133340783293,173.985485069079));
#45067=CARTESIAN_POINT('Origin',(-51.2438457370578,57.3835762739523,173.985485069079));
#45068=CARTESIAN_POINT('Ctrl Pts',(-49.676843289894,59.3614282330636,172.857169043842));
#45069=CARTESIAN_POINT('Ctrl Pts',(-49.6580501443528,59.498785825288,172.940667815898));
#45070=CARTESIAN_POINT('Ctrl Pts',(-49.5614006736427,59.5779430613272,173.043611870202));
#45071=CARTESIAN_POINT('Ctrl Pts',(-49.8129218697063,59.2066852860614,173.020976119607));
#45072=CARTESIAN_POINT('Ctrl Pts',(-49.8268191099127,59.3595810228937,173.140746393147));
#45073=CARTESIAN_POINT('Ctrl Pts',(-49.7298982507317,59.4401605537898,173.288593641521));
#45074=CARTESIAN_POINT('Ctrl Pts',(-49.9751587473744,59.0175746776917,173.132009583873));
#45075=CARTESIAN_POINT('Ctrl Pts',(-50.0283787246662,59.1891576068682,173.26617245629));
#45076=CARTESIAN_POINT('Ctrl Pts',(-49.9342084666479,59.2692635558937,173.455528336301));
#45077=CARTESIAN_POINT('Ctrl Pts',(-50.2670349607775,58.6648561595715,173.282713630629));
#45078=CARTESIAN_POINT('Ctrl Pts',(-50.3867087288933,58.8763902547733,173.422336146559));
#45079=CARTESIAN_POINT('Ctrl Pts',(-50.3068160600608,58.946637106271,173.681583012477));
#45080=CARTESIAN_POINT('Ctrl Pts',(-50.3913565197452,58.5110970032596,173.331875725947));
#45081=CARTESIAN_POINT('Ctrl Pts',(-50.5416645611132,58.7381013798362,173.467425863685));
#45082=CARTESIAN_POINT('Ctrl Pts',(-50.4671147462085,58.8047920444951,173.755313568593));
#45083=CARTESIAN_POINT('Ctrl Pts',(-50.8097833774366,57.9804901848007,173.46326053759));
#45084=CARTESIAN_POINT('Ctrl Pts',(-51.0806778350923,58.2463716358246,173.571501704738));
#45085=CARTESIAN_POINT('Ctrl Pts',(-51.0122898852652,58.3106471527106,173.952327305448));
#45086=CARTESIAN_POINT('Ctrl Pts',(-51.1047582211487,57.5839691659291,173.498876066328));
#45087=CARTESIAN_POINT('Ctrl Pts',(-51.4575793662449,57.881015208655,173.541235698465));
#45088=CARTESIAN_POINT('Ctrl Pts',(-51.4062439592343,57.9336438396564,174.005637220798));
#45089=CARTESIAN_POINT('Ctrl Pts',(-51.3846028209176,57.183358971478,173.481037601188));
#45090=CARTESIAN_POINT('Ctrl Pts',(-51.7691525391572,57.5641765559212,173.436036324449));
#45091=CARTESIAN_POINT('Ctrl Pts',(-51.7892845019502,57.5437998061236,173.978750519954));
#45092=CARTESIAN_POINT('Origin',(-49.394587641375,59.0674820360207,173.235485069079));
#45093=CARTESIAN_POINT('Ctrl Pts',(-49.7140665684645,59.4521029079787,173.235485069079));
#45094=CARTESIAN_POINT('Ctrl Pts',(-49.8076683737025,59.3743541260188,173.092919514947));
#45095=CARTESIAN_POINT('Ctrl Pts',(-49.7994785223376,59.2209856988867,172.985485069079));
#45096=CARTESIAN_POINT('Ctrl Pts',(-49.3244877069872,59.7757001065599,172.810949602497));
#45097=CARTESIAN_POINT('Ctrl Pts',(-49.4175936181462,59.7012196303848,172.669550113054));
#45098=CARTESIAN_POINT('Ctrl Pts',(-49.4120033989242,59.551605021816,172.560949601135));
#45099=CARTESIAN_POINT('Ctrl Pts',(-48.9215898703068,60.0925595649752,172.396514721378));
#45100=CARTESIAN_POINT('Ctrl Pts',(-49.0132975775448,60.0219725953743,172.255650553252));
#45101=CARTESIAN_POINT('Ctrl Pts',(-49.0106022401066,59.8760222809677,172.146514351631));
#45102=CARTESIAN_POINT('Ctrl Pts',(-48.5031673671099,60.4028926537974,171.994932980254));
#45103=CARTESIAN_POINT('Ctrl Pts',(-48.5921091241355,60.3369268656953,171.853849669263));
#45104=CARTESIAN_POINT('Ctrl Pts',(-48.5928620772033,60.1944375331114,171.744932980254));
#45105=CARTESIAN_POINT('Origin',(-37.6267629804773,17.3035841126903,177.985485069079));
#45106=CARTESIAN_POINT('Origin',(-39.8623336503921,1.96564996953346,177.985485069079));
#45107=CARTESIAN_POINT('Origin',(-52.0389027942237,11.5991800255814,177.985485069079));
#45108=CARTESIAN_POINT('Origin',(-55.2932569457149,10.3110887801052,177.985485069079));
#45109=CARTESIAN_POINT('Origin',(-56.6916004724222,13.5196142017461,177.985485069079));
#45110=CARTESIAN_POINT('Origin',(-67.58190263219,8.77338921431569,177.985485069079));
#45111=CARTESIAN_POINT('Origin',(-94.0351308638859,47.8471884530858,177.985485069079));
#45112=CARTESIAN_POINT('Origin',(-58.9792278552929,42.2495403530246,177.985485069079));
#45113=CARTESIAN_POINT('Origin',(-31.8232466514532,37.9133340783293,177.985485069079));
#45114=CARTESIAN_POINT('Origin',(-51.243845737057,57.3835762739531,177.985485069079));
#45115=CARTESIAN_POINT('Ctrl Pts',(-51.3851747440281,57.1830027074348,178.489845032705));
#45116=CARTESIAN_POINT('Ctrl Pts',(-51.7698287477023,57.5635493714596,178.53459520218));
#45117=CARTESIAN_POINT('Ctrl Pts',(-51.789795174837,57.5433312673965,177.992059147256));
#45118=CARTESIAN_POINT('Ctrl Pts',(-51.1036551824481,57.5857370375821,178.47242911223));
#45119=CARTESIAN_POINT('Ctrl Pts',(-51.4556422663022,57.882802074248,178.429816451876));
#45120=CARTESIAN_POINT('Ctrl Pts',(-51.4046161396593,57.9351319791878,177.965865526389));
#45121=CARTESIAN_POINT('Ctrl Pts',(-50.812871026537,57.9768655506053,178.506778396529));
#45122=CARTESIAN_POINT('Ctrl Pts',(-51.0847171506893,58.2426715965213,178.398610314328));
#45123=CARTESIAN_POINT('Ctrl Pts',(-51.0161416619809,58.3071396903623,178.017328502921));
#45124=CARTESIAN_POINT('Ctrl Pts',(-50.39072672801,58.5121320105389,178.639222923132));
#45125=CARTESIAN_POINT('Ctrl Pts',(-50.5408096374063,58.7388868900845,178.503564579484));
#45126=CARTESIAN_POINT('Ctrl Pts',(-50.4661837565912,58.8056426366741,178.215960736115));
#45127=CARTESIAN_POINT('Ctrl Pts',(-50.2654292154088,58.6670064325193,178.688993669122));
#45128=CARTESIAN_POINT('Ctrl Pts',(-50.384555500579,58.8782789036964,178.549394330658));
#45129=CARTESIAN_POINT('Ctrl Pts',(-50.3046760179673,58.9484994170746,178.29061015284));
#45130=CARTESIAN_POINT('Ctrl Pts',(-49.9761487934086,59.0165015159078,178.838454681089));
#45131=CARTESIAN_POINT('Ctrl Pts',(-50.0294357633358,59.1882221141344,178.704350540701));
#45132=CARTESIAN_POINT('Ctrl Pts',(-49.9354391713799,59.2681848187678,178.514801007031));
#45133=CARTESIAN_POINT('Ctrl Pts',(-49.8137887158582,59.2058315816185,178.948821207635));
#45134=CARTESIAN_POINT('Ctrl Pts',(-49.8279315490083,59.358683921035,178.828773746461));
#45135=CARTESIAN_POINT('Ctrl Pts',(-49.7309210947959,59.4393519811699,178.680758434674));
#45136=CARTESIAN_POINT('Ctrl Pts',(-49.6753781533107,59.3631653373938,179.115257436673));
#45137=CARTESIAN_POINT('Ctrl Pts',(-49.6562522395083,59.5002721847792,179.032027213671));
#45138=CARTESIAN_POINT('Ctrl Pts',(-49.5596295986081,59.5793903823432,178.92957895201));
#45139=CARTESIAN_POINT('Origin',(-49.3945876413725,59.0674820360227,178.735485069082));
#45140=CARTESIAN_POINT('Ctrl Pts',(-49.7994785223352,59.2209856988888,178.985485069082));
#45141=CARTESIAN_POINT('Ctrl Pts',(-49.8076683737,59.3743541260209,178.878050623215));
#45142=CARTESIAN_POINT('Ctrl Pts',(-49.714066568462,59.4521029079807,178.735485069082));
#45143=CARTESIAN_POINT('Ctrl Pts',(-49.412003398922,59.5516050218084,179.410020537031));
#45144=CARTESIAN_POINT('Ctrl Pts',(-49.4175936181378,59.7012196303778,179.301420025102));
#45145=CARTESIAN_POINT('Ctrl Pts',(-49.3244877069919,59.775700106556,179.16002053567));
#45146=CARTESIAN_POINT('Ctrl Pts',(-49.0106022401058,59.8760222809537,179.824455786539));
#45147=CARTESIAN_POINT('Ctrl Pts',(-49.0132975775679,60.0219725953311,179.715319584971));
#45148=CARTESIAN_POINT('Ctrl Pts',(-48.9215898703156,60.0925595649687,179.5744554168));
#45149=CARTESIAN_POINT('Ctrl Pts',(-48.5928620772034,60.1944375331114,180.226037157904));
#45150=CARTESIAN_POINT('Ctrl Pts',(-48.5921091241356,60.3369268656953,180.117120468896));
#45151=CARTESIAN_POINT('Ctrl Pts',(-48.5031673671099,60.4028926537974,179.976037157904));
#45152=CARTESIAN_POINT('Ctrl Pts',(-45.4569991048231,35.0869155900178,172.985485069079));
#45153=CARTESIAN_POINT('Ctrl Pts',(-44.9016339249302,35.0941792779979,172.955802932359));
#45154=CARTESIAN_POINT('Ctrl Pts',(-44.9520576904499,35.5723002038223,173.235485069079));
#45155=CARTESIAN_POINT('Ctrl Pts',(-45.4850941496413,35.3295082190528,172.566233948071));
#45156=CARTESIAN_POINT('Ctrl Pts',(-44.9281468509024,35.3344337427825,172.534956661662));
#45157=CARTESIAN_POINT('Ctrl Pts',(-44.9775100896269,35.8136412566676,172.81623419061));
#45158=CARTESIAN_POINT('Ctrl Pts',(-45.5125916761024,35.5723252360281,172.14705466709));
#45159=CARTESIAN_POINT('Ctrl Pts',(-44.9537495963942,35.5744329169919,172.114352981929));
#45160=CARTESIAN_POINT('Ctrl Pts',(-45.0020952646643,36.0551804790105,172.397054925059));
#45161=CARTESIAN_POINT('Ctrl Pts',(-45.5396570323393,35.815459379751,171.727986820601));
#45162=CARTESIAN_POINT('Ctrl Pts',(-44.9783867312583,35.8135096162751,171.694926243495));
#45163=CARTESIAN_POINT('Ctrl Pts',(-45.0258168897239,36.2969847903722,171.977986820601));
#45164=CARTESIAN_POINT('Origin',(-45.4493000945566,35.5198598419035,173.235485069079));
#45165=CARTESIAN_POINT('Ctrl Pts',(-45.3036829175493,34.2202360714903,173.485485069079));
#45166=CARTESIAN_POINT('Ctrl Pts',(-44.8071649770098,34.2791422233116,173.485485069079));
#45167=CARTESIAN_POINT('Ctrl Pts',(-44.8071649770098,34.2791422233116,173.985485069079));
#45168=CARTESIAN_POINT('Ctrl Pts',(-45.3338963953346,34.3940443299001,173.485485069079));
#45169=CARTESIAN_POINT('Ctrl Pts',(-44.8279831491234,34.4546178863727,173.475857632828));
#45170=CARTESIAN_POINT('Ctrl Pts',(-44.8379572766539,34.538689464662,173.985485049617));
#45171=CARTESIAN_POINT('Ctrl Pts',(-45.3644831092931,34.5691582546223,173.438504175172));
#45172=CARTESIAN_POINT('Ctrl Pts',(-44.84765733035,34.6236472660135,173.417377867645));
#45173=CARTESIAN_POINT('Ctrl Pts',(-44.8678394640859,34.800067602205,173.915013729195));
#45174=CARTESIAN_POINT('Ctrl Pts',(-45.4044745628099,34.7951467101956,173.308260039551));
#45175=CARTESIAN_POINT('Ctrl Pts',(-44.8718806226984,34.8337506678808,173.278188236865));
#45176=CARTESIAN_POINT('Ctrl Pts',(-44.9052767643286,35.1372390952084,173.719647524298));
#45177=CARTESIAN_POINT('Ctrl Pts',(-45.417105936473,34.8659857778945,173.254031151206));
#45178=CARTESIAN_POINT('Ctrl Pts',(-44.8792949307336,34.898439442477,173.2217377076));
#45179=CARTESIAN_POINT('Ctrl Pts',(-44.9168097068416,35.2429009650579,173.638304190863));
#45180=CARTESIAN_POINT('Ctrl Pts',(-45.4392598534242,34.9893244322491,173.130935739704));
#45181=CARTESIAN_POINT('Ctrl Pts',(-44.8919644948922,35.0092694227254,173.097445835965));
#45182=CARTESIAN_POINT('Ctrl Pts',(-44.9366510910588,35.4268263152626,173.453661076422));
#45183=CARTESIAN_POINT('Ctrl Pts',(-45.4489103970047,35.042562611079,173.062045438043));
#45184=CARTESIAN_POINT('Ctrl Pts',(-44.8972783322719,35.0559155097348,173.029495931902));
#45185=CARTESIAN_POINT('Ctrl Pts',(-44.9450858967755,35.5061932716661,173.35032414664));
#45186=CARTESIAN_POINT('Ctrl Pts',(-45.4569991048231,35.0869155900178,172.985485069079));
#45187=CARTESIAN_POINT('Ctrl Pts',(-44.9016339249302,35.0941792779979,172.955802932359));
#45188=CARTESIAN_POINT('Ctrl Pts',(-44.9520576904499,35.5723002038223,173.235485069079));
#45189=CARTESIAN_POINT('Origin',(-45.3036829175493,34.2202360714903,173.985485069079));
#45190=CARTESIAN_POINT('Origin',(54.4964231308939,46.060372587574,173.985485069079));
#45191=CARTESIAN_POINT('Origin',(-43.2773451499467,22.8108513846653,173.985485069079));
#45192=CARTESIAN_POINT('Origin',(-31.1164286971058,25.7025828775644,173.985485069079));
#45193=CARTESIAN_POINT('Origin',(-36.2883138077383,14.3227057076466,173.985485069079));
#45194=CARTESIAN_POINT('Origin',(-38.9776940652673,8.40516957928931,173.985485069079));
#45195=CARTESIAN_POINT('Origin',(-39.8623336503921,1.96564996953346,173.985485069079));
#45196=CARTESIAN_POINT('Origin',(-39.8623336503921,1.96564996953345,173.985485069079));
#45197=CARTESIAN_POINT('Origin',(-39.8623336503921,1.96564996953346,173.985485069079));
#45198=CARTESIAN_POINT('Origin',(-39.8623336503921,1.96564996953346,178.485485069079));
#45199=CARTESIAN_POINT('Origin',(-39.8623336503921,1.96564996953346,177.985485069079));
#45200=CARTESIAN_POINT('Origin',(-39.8623336503921,1.96564996953345,177.985485069079));
#45201=CARTESIAN_POINT('Origin',(-39.8623336503921,1.96564996953346,177.985485069079));
#45202=CARTESIAN_POINT('Origin',(-38.9776940652673,8.40516957928931,177.985485069079));
#45203=CARTESIAN_POINT('Origin',(-36.2883138077383,14.3227057076466,177.985485069079));
#45204=CARTESIAN_POINT('Origin',(-31.1164286971058,25.7025828775644,177.985485069079));
#45205=CARTESIAN_POINT('Origin',(-43.2773451499467,22.8108513846653,177.985485069079));
#45206=CARTESIAN_POINT('Origin',(54.4964231308939,46.060372587574,177.985485069079));
#45207=CARTESIAN_POINT('Origin',(-45.3036829175493,34.2202360714903,177.985485069079));
#45208=CARTESIAN_POINT('Ctrl Pts',(-45.4569991048231,35.0869155900178,178.985485069079));
#45209=CARTESIAN_POINT('Ctrl Pts',(-44.9016339249302,35.0941792779979,179.0151672058));
#45210=CARTESIAN_POINT('Ctrl Pts',(-44.9520576904499,35.5723002038223,178.735485069079));
#45211=CARTESIAN_POINT('Ctrl Pts',(-45.4410006746859,34.9991910657925,178.83405844334));
#45212=CARTESIAN_POINT('Ctrl Pts',(-44.8930599489135,35.0188571214058,178.870102671035));
#45213=CARTESIAN_POINT('Ctrl Pts',(-44.9382677607559,35.4415433298683,178.508337952365));
#45214=CARTESIAN_POINT('Ctrl Pts',(-45.4177353589643,34.8700866935674,178.705789670185));
#45215=CARTESIAN_POINT('Ctrl Pts',(-44.8800761442588,34.9048322093886,178.739759632446));
#45216=CARTESIAN_POINT('Ctrl Pts',(-44.9176930036587,35.2490486968859,178.315941970112));
#45217=CARTESIAN_POINT('Ctrl Pts',(-45.3777210193303,34.6439624480249,178.575633526873));
#45218=CARTESIAN_POINT('Ctrl Pts',(-44.8555949763002,34.6924969087779,178.599259564719));
#45219=CARTESIAN_POINT('Ctrl Pts',(-44.8802307081201,34.9116742540591,178.120707756082));
#45220=CARTESIAN_POINT('Ctrl Pts',(-45.3632480720711,34.5616383925205,178.541657619885));
#45221=CARTESIAN_POINT('Ctrl Pts',(-44.8465284950399,34.6142452624173,178.560861887554));
#45222=CARTESIAN_POINT('Ctrl Pts',(-44.8663865052777,34.7888188171875,178.069743897378));
#45223=CARTESIAN_POINT('Ctrl Pts',(-45.3339158795757,34.3939812335556,178.496912907544));
#45224=CARTESIAN_POINT('Ctrl Pts',(-44.8275659262796,34.4518581195231,178.506832300477));
#45225=CARTESIAN_POINT('Ctrl Pts',(-44.8376784522628,34.5385617116783,178.002626824687));
#45226=CARTESIAN_POINT('Ctrl Pts',(-45.3189633638158,34.3081394824255,178.485485069079));
#45227=CARTESIAN_POINT('Ctrl Pts',(-44.8176339640159,34.3673849580269,178.490326489291));
#45228=CARTESIAN_POINT('Ctrl Pts',(-44.8227374568447,34.4104021236386,177.985485079905));
#45229=CARTESIAN_POINT('Ctrl Pts',(-45.3036829175493,34.2202360714903,178.485485069079));
#45230=CARTESIAN_POINT('Ctrl Pts',(-44.8071649770098,34.2791422233116,178.485485069079));
#45231=CARTESIAN_POINT('Ctrl Pts',(-44.8071649770098,34.2791422233116,177.985485069079));
#45232=CARTESIAN_POINT('Origin',(-45.4493000945566,35.5198598419035,178.735485069079));
#45233=CARTESIAN_POINT('Ctrl Pts',(-44.9520576904499,35.5723002038223,178.735485069079));
#45234=CARTESIAN_POINT('Ctrl Pts',(-44.9016339249302,35.0941792779979,179.0151672058));
#45235=CARTESIAN_POINT('Ctrl Pts',(-45.4569991048231,35.0869155900178,178.985485069079));
#45236=CARTESIAN_POINT('Ctrl Pts',(-44.9775100896269,35.8136412566674,179.154735947548));
#45237=CARTESIAN_POINT('Ctrl Pts',(-44.928146850906,35.334433742785,179.436013476495));
#45238=CARTESIAN_POINT('Ctrl Pts',(-45.4850941496413,35.3295082190525,179.404736190087));
#45239=CARTESIAN_POINT('Ctrl Pts',(-45.0020952646649,36.0551804790164,179.573915213096));
#45240=CARTESIAN_POINT('Ctrl Pts',(-44.9537495963754,35.5744329169963,179.856617156227));
#45241=CARTESIAN_POINT('Ctrl Pts',(-45.5125916761142,35.572325236028,179.823915471068));
#45242=CARTESIAN_POINT('Ctrl Pts',(-45.0258168897239,36.296984790372,179.992983317557));
#45243=CARTESIAN_POINT('Ctrl Pts',(-44.9783867312583,35.8135096162749,180.276043894663));
#45244=CARTESIAN_POINT('Ctrl Pts',(-45.5396570323393,35.8154593797507,180.242983317557));
#47697=UNCERTAINTY_MEASURE_WITH_UNIT(LENGTH_MEASURE(0.01),#47718,
'DISTANCE_ACCURACY_VALUE',
'Maximum model space distance between geometric entities at asserted c
onnectivities');
#47703=UNCERTAINTY_MEASURE_WITH_UNIT(LENGTH_MEASURE(0.01),#47718,
'DISTANCE_ACCURACY_VALUE',
'Maximum model space distance between geometric entities at asserted c
onnectivities');
#47711=(
GEOMETRIC_REPRESENTATION_CONTEXT(3)
GLOBAL_UNCERTAINTY_ASSIGNED_CONTEXT((#47697))
GLOBAL_UNIT_ASSIGNED_CONTEXT((#47718,#47720,#47721))
REPRESENTATION_CONTEXT('','3D')
);
#47717=(
GEOMETRIC_REPRESENTATION_CONTEXT(3)
GLOBAL_UNCERTAINTY_ASSIGNED_CONTEXT((#47703))
GLOBAL_UNIT_ASSIGNED_CONTEXT((#47718,#47720,#47721))
REPRESENTATION_CONTEXT('','3D')
);
#47718=(
LENGTH_UNIT()
NAMED_UNIT(*)
SI_UNIT(.MILLI.,.METRE.)
);
#47720=(
NAMED_UNIT(*)
PLANE_ANGLE_UNIT()
SI_UNIT($,.RADIAN.)
);
#47721=(
NAMED_UNIT(*)
SI_UNIT($,.STERADIAN.)
SOLID_ANGLE_UNIT()
);
#47729=SHAPE_DEFINITION_REPRESENTATION(#47742,#47767);
#47742=PRODUCT_DEFINITION_SHAPE('',$,#47781);
#47767=SHAPE_REPRESENTATION('',(#9515),#47711);
#47773=PRODUCT_DEFINITION_CONTEXT('part definition',#47814,'design');
#47781=PRODUCT_DEFINITION('Movable Jaw','Movable Jaw',#47794,#47773);
#47794=PRODUCT_DEFINITION_FORMATION('',$,#47823);
#47814=APPLICATION_CONTEXT(
'Core Data for Automotive Mechanical Design Process');
#47815=PRODUCT_CONTEXT('part definition',#47814,'mechanical');
#47823=PRODUCT('Movable Jaw','Movable Jaw',$,(#47815));
#47830=PRESENTATION_STYLE_ASSIGNMENT((#47832));
#47832=SURFACE_STYLE_USAGE(.BOTH.,#47834);
#47834=SURFACE_SIDE_STYLE('',(#47836));
#47836=SURFACE_STYLE_FILL_AREA(#47838);
#47838=FILL_AREA_STYLE('Opaque(202,209,238)',(#47840));
#47840=FILL_AREA_STYLE_COLOUR('Opaque(202,209,238)',#47842);
#47842=COLOUR_RGB('Opaque(202,209,238)', 0.66274510, 0.83137255, 0.94901961);
ENDSEC;
END-ISO-10303-21;
